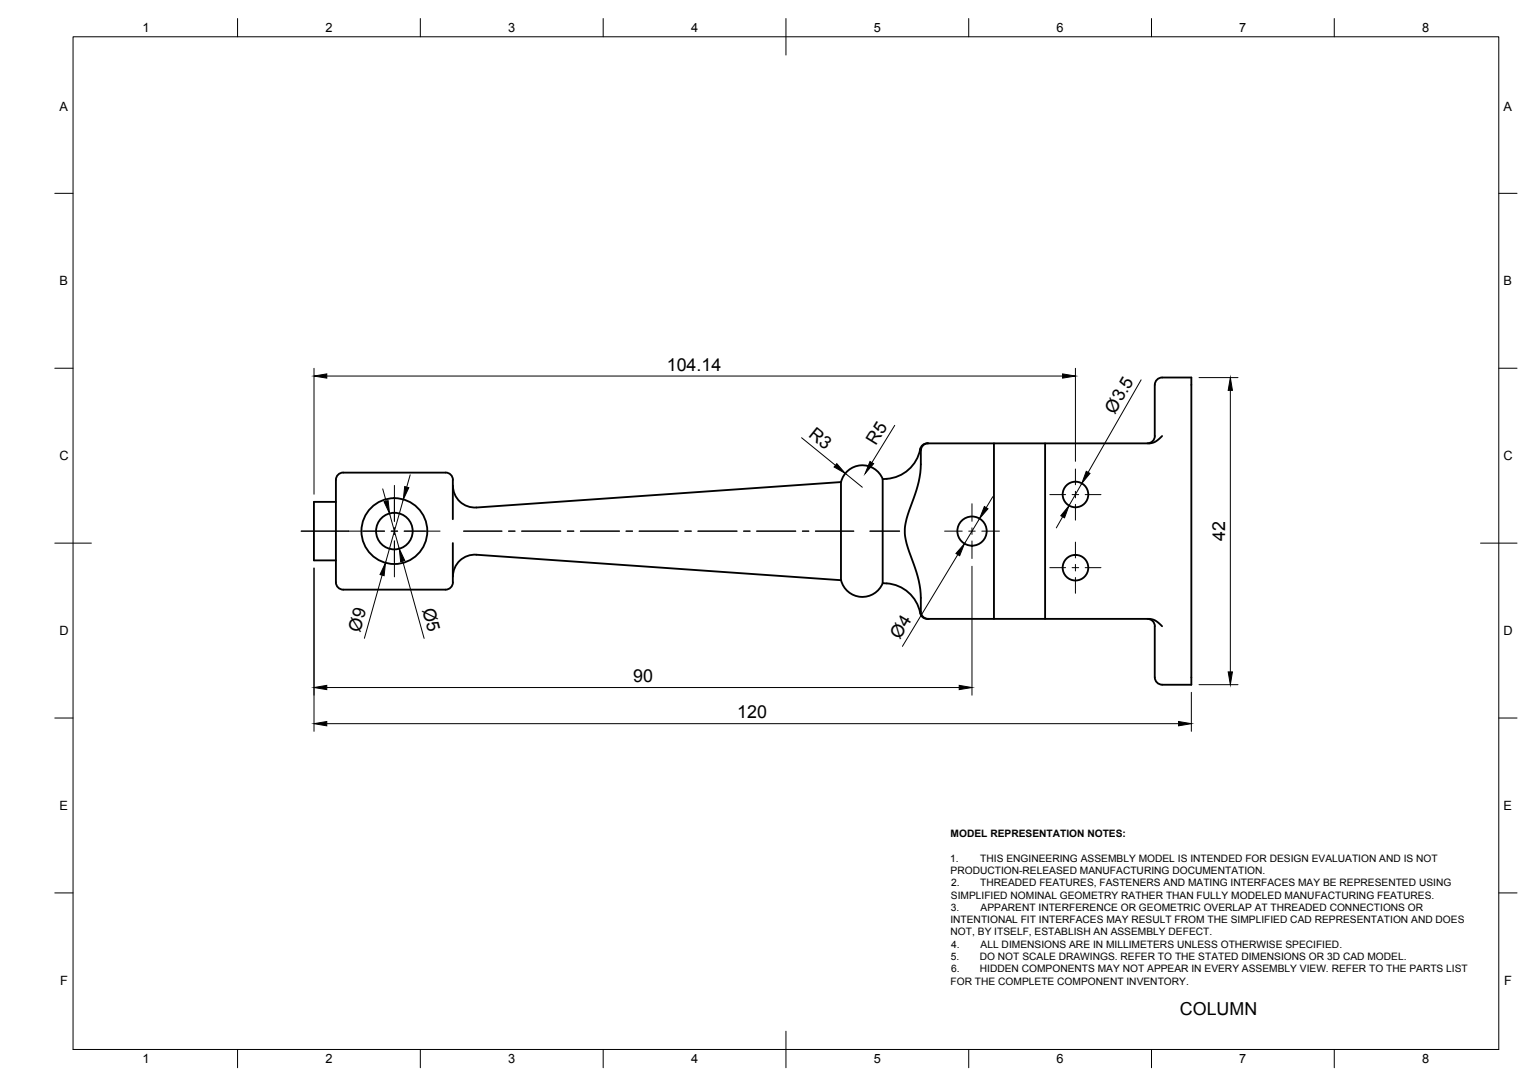
ISO-10303-21;
HEADER;
/* Generated by software containing ST-Developer
 * from STEP Tools, Inc. (www.steptools.com) 
 */

FILE_DESCRIPTION(
/* description */ (''),
/* implementation_level */ '2;1');

FILE_NAME(
/* name */ 'COLUMN.step',
/* time_stamp */ '2026-10-06T01:16:10-07:00',
/* author */ (''),
/* organization */ (''),
/* preprocessor_version */ 'ST-DEVELOPER v20.2',
/* originating_system */ 'Autodesk Translation Framework v15.15.0.0',
/* authorisation */ '');

FILE_SCHEMA (('AUTOMOTIVE_DESIGN { 1 0 10303 214 3 1 1 }'));
ENDSEC;

DATA;
#10=MECHANICAL_DESIGN_GEOMETRIC_PRESENTATION_REPRESENTATION('',(#300,#301,#302),#17113);
#105=ELLIPSE('',#6445,1.4142135623731,1.);
#106=ELLIPSE('',#6457,1.41421356237309,1.);
#109=(
BOUNDED_SURFACE()
B_SPLINE_SURFACE(3,3,((#9243,#9244,#9245,#9246,#9247,#9248,#9249,#9250,
#9251,#9252,#9253,#9254,#9255),(#9256,#9257,#9258,#9259,#9260,#9261,#9262,
#9263,#9264,#9265,#9266,#9267,#9268),(#9269,#9270,#9271,#9272,#9273,#9274,
#9275,#9276,#9277,#9278,#9279,#9280,#9281),(#9282,#9283,#9284,#9285,#9286,
#9287,#9288,#9289,#9290,#9291,#9292,#9293,#9294)),.UNSPECIFIED.,.F.,.F.,
 .F.)
B_SPLINE_SURFACE_WITH_KNOTS((4,4),(4,1,1,1,1,1,1,1,1,1,4),(0.,1.),(-0.01854087386661,
0.,0.124538046056,0.2354380828125,0.3411963661322,0.4510248812945,0.5701285898783,
0.7002368466242,0.8429884965965,1.,1.018551127109),.UNSPECIFIED.)
GEOMETRIC_REPRESENTATION_ITEM()
RATIONAL_B_SPLINE_SURFACE(((1.236576476327,1.236576476327,1.236576476327,
1.236576476327,1.236576476327,1.236576476327,1.236576476327,1.236576476327,
1.236576476327,1.236576476327,1.236576476327,1.236576476327,1.236576476327),
(0.9211411745578,0.9211411745578,0.9211411745578,0.9211411745578,0.9211411745578,
0.9211411745578,0.9211411745578,0.9211411745578,0.9211411745578,0.9211411745578,
0.9211411745578,0.9211411745578,0.9211411745578),(0.9211411745578,0.9211411745578,
0.9211411745578,0.9211411745578,0.9211411745578,0.9211411745578,0.9211411745578,
0.9211411745578,0.9211411745578,0.9211411745578,0.9211411745578,0.9211411745578,
0.9211411745578),(1.236576476327,1.236576476327,1.236576476327,1.236576476327,
1.236576476327,1.236576476327,1.236576476327,1.236576476327,1.236576476327,
1.236576476327,1.236576476327,1.236576476327,1.236576476327)))
REPRESENTATION_ITEM('')
SURFACE()
);
#110=(
BOUNDED_SURFACE()
B_SPLINE_SURFACE(3,3,((#9423,#9424,#9425,#9426,#9427,#9428,#9429,#9430,
#9431,#9432,#9433,#9434,#9435),(#9436,#9437,#9438,#9439,#9440,#9441,#9442,
#9443,#9444,#9445,#9446,#9447,#9448),(#9449,#9450,#9451,#9452,#9453,#9454,
#9455,#9456,#9457,#9458,#9459,#9460,#9461),(#9462,#9463,#9464,#9465,#9466,
#9467,#9468,#9469,#9470,#9471,#9472,#9473,#9474)),.UNSPECIFIED.,.F.,.F.,
 .F.)
B_SPLINE_SURFACE_WITH_KNOTS((4,4),(4,1,1,1,1,1,1,1,1,1,4),(0.,1.),(-0.01854087386661,
0.,0.124538046056,0.2354380828125,0.3411963661322,0.4510248812945,0.5701285898783,
0.7002368466242,0.8429884965965,1.,1.018551127109),.UNSPECIFIED.)
GEOMETRIC_REPRESENTATION_ITEM()
RATIONAL_B_SPLINE_SURFACE(((1.236576476327,1.236576476327,1.236576476327,
1.236576476327,1.236576476327,1.236576476327,1.236576476327,1.236576476327,
1.236576476327,1.236576476327,1.236576476327,1.236576476327,1.236576476327),
(0.9211411745578,0.9211411745578,0.9211411745578,0.9211411745578,0.9211411745578,
0.9211411745578,0.9211411745578,0.9211411745578,0.9211411745578,0.9211411745578,
0.9211411745578,0.9211411745578,0.9211411745578),(0.9211411745578,0.9211411745578,
0.9211411745578,0.9211411745578,0.9211411745578,0.9211411745578,0.9211411745578,
0.9211411745578,0.9211411745578,0.9211411745578,0.9211411745578,0.9211411745578,
0.9211411745578),(1.236576476327,1.236576476327,1.236576476327,1.236576476327,
1.236576476327,1.236576476327,1.236576476327,1.236576476327,1.236576476327,
1.236576476327,1.236576476327,1.236576476327,1.236576476327)))
REPRESENTATION_ITEM('')
SURFACE()
);
#111=(
BOUNDED_SURFACE()
B_SPLINE_SURFACE(3,3,((#9791,#9792,#9793,#9794,#9795,#9796,#9797,#9798,
#9799,#9800,#9801,#9802,#9803,#9804,#9805,#9806,#9807),(#9808,#9809,#9810,
#9811,#9812,#9813,#9814,#9815,#9816,#9817,#9818,#9819,#9820,#9821,#9822,
#9823,#9824),(#9825,#9826,#9827,#9828,#9829,#9830,#9831,#9832,#9833,#9834,
#9835,#9836,#9837,#9838,#9839,#9840,#9841),(#9842,#9843,#9844,#9845,#9846,
#9847,#9848,#9849,#9850,#9851,#9852,#9853,#9854,#9855,#9856,#9857,#9858)),
 .UNSPECIFIED.,.F.,.F.,.F.)
B_SPLINE_SURFACE_WITH_KNOTS((4,4),(4,1,1,1,1,1,1,1,1,1,1,1,1,1,4),(0.,1.),
(-0.009903506240665,0.,0.09441816002876,0.1881578788494,0.280939071815,
0.3715247502583,0.4641517260557,0.5619785611963,0.6570408645664,0.7414898315922,
0.8160167895793,0.8826179898193,0.9432826185749,1.,1.009908876933),
 .UNSPECIFIED.)
GEOMETRIC_REPRESENTATION_ITEM()
RATIONAL_B_SPLINE_SURFACE(((1.236576619558,1.236576619558,1.236576619558,
1.236576619558,1.236576619558,1.236576619558,1.236576619558,1.236576619558,
1.236576619558,1.236576619558,1.236576619558,1.236576619558,1.236576619558,
1.236576619558,1.236576619558,1.236576619558,1.236576619558),(0.9211411268139,
0.9211411268139,0.9211411268139,0.9211411268139,0.9211411268139,0.9211411268139,
0.9211411268139,0.9211411268139,0.9211411268139,0.9211411268139,0.9211411268139,
0.9211411268139,0.9211411268139,0.9211411268139,0.9211411268139,0.9211411268139,
0.9211411268139),(0.9211411268139,0.9211411268139,0.9211411268139,0.9211411268139,
0.9211411268139,0.9211411268139,0.9211411268139,0.9211411268139,0.9211411268139,
0.9211411268139,0.9211411268139,0.9211411268139,0.9211411268139,0.9211411268139,
0.9211411268139,0.9211411268139,0.9211411268139),(1.236576619558,1.236576619558,
1.236576619558,1.236576619558,1.236576619558,1.236576619558,1.236576619558,
1.236576619558,1.236576619558,1.236576619558,1.236576619558,1.236576619558,
1.236576619558,1.236576619558,1.236576619558,1.236576619558,1.236576619558)))
REPRESENTATION_ITEM('')
SURFACE()
);
#112=(
BOUNDED_SURFACE()
B_SPLINE_SURFACE(3,3,((#10155,#10156,#10157,#10158,#10159,#10160,#10161,
#10162,#10163,#10164,#10165),(#10166,#10167,#10168,#10169,#10170,#10171,
#10172,#10173,#10174,#10175,#10176),(#10177,#10178,#10179,#10180,#10181,
#10182,#10183,#10184,#10185,#10186,#10187),(#10188,#10189,#10190,#10191,
#10192,#10193,#10194,#10195,#10196,#10197,#10198)),.UNSPECIFIED.,.F.,.F.,
 .F.)
B_SPLINE_SURFACE_WITH_KNOTS((4,4),(4,1,1,1,1,1,1,1,4),(0.,1.),(-0.0117961357116,
0.,0.1633770608974,0.3160773256608,0.4701362865974,0.6315432333968,0.8054144885927,
1.,1.011975292336),.UNSPECIFIED.)
GEOMETRIC_REPRESENTATION_ITEM()
RATIONAL_B_SPLINE_SURFACE(((1.236576493506,1.236576493506,1.236576493506,
1.236576493506,1.236576493506,1.236576493506,1.236576493506,1.236576493506,
1.236576493506,1.236576493506,1.236576493506),(0.9211411688312,0.9211411688312,
0.9211411688312,0.9211411688312,0.9211411688312,0.9211411688312,0.9211411688312,
0.9211411688312,0.9211411688312,0.9211411688312,0.9211411688312),(0.9211411688312,
0.9211411688312,0.9211411688312,0.9211411688312,0.9211411688312,0.9211411688312,
0.9211411688312,0.9211411688312,0.9211411688312,0.9211411688312,0.9211411688312),
(1.236576493506,1.236576493506,1.236576493506,1.236576493506,1.236576493506,
1.236576493506,1.236576493506,1.236576493506,1.236576493506,1.236576493506,
1.236576493506)))
REPRESENTATION_ITEM('')
SURFACE()
);
#113=(
BOUNDED_SURFACE()
B_SPLINE_SURFACE(3,3,((#10200,#10201,#10202,#10203,#10204,#10205,#10206,
#10207,#10208,#10209,#10210,#10211,#10212),(#10213,#10214,#10215,#10216,
#10217,#10218,#10219,#10220,#10221,#10222,#10223,#10224,#10225),(#10226,
#10227,#10228,#10229,#10230,#10231,#10232,#10233,#10234,#10235,#10236,#10237,
#10238),(#10239,#10240,#10241,#10242,#10243,#10244,#10245,#10246,#10247,
#10248,#10249,#10250,#10251)),.UNSPECIFIED.,.F.,.F.,.F.)
B_SPLINE_SURFACE_WITH_KNOTS((4,4),(4,1,1,1,1,1,1,1,1,1,4),(0.,1.),(-0.02387271189713,
0.,0.1233219598256,0.2447228034141,0.3668475159477,0.4855515195745,0.6022629448181,
0.7239422574426,0.8555602069799,1.,1.011825585123),.UNSPECIFIED.)
GEOMETRIC_REPRESENTATION_ITEM()
RATIONAL_B_SPLINE_SURFACE(((1.236576471212,1.236576471212,1.236576471212,
1.236576471212,1.236576471212,1.236576471212,1.236576471212,1.236576471212,
1.236576471212,1.236576471212,1.236576471212,1.236576471212,1.236576471212),
(0.9211411762628,0.9211411762628,0.9211411762628,0.9211411762628,0.9211411762628,
0.9211411762628,0.9211411762628,0.9211411762628,0.9211411762628,0.9211411762628,
0.9211411762628,0.9211411762628,0.9211411762628),(0.9211411762628,0.9211411762628,
0.9211411762628,0.9211411762628,0.9211411762628,0.9211411762628,0.9211411762628,
0.9211411762628,0.9211411762628,0.9211411762628,0.9211411762628,0.9211411762628,
0.9211411762628),(1.236576471212,1.236576471212,1.236576471212,1.236576471212,
1.236576471212,1.236576471212,1.236576471212,1.236576471212,1.236576471212,
1.236576471212,1.236576471212,1.236576471212,1.236576471212)))
REPRESENTATION_ITEM('')
SURFACE()
);
#114=SPHERICAL_SURFACE('',#6330,1.);
#115=SPHERICAL_SURFACE('',#6351,1.);
#116=SPHERICAL_SURFACE('',#6354,1.);
#117=SPHERICAL_SURFACE('',#6359,1.);
#118=SPHERICAL_SURFACE('',#6367,1.);
#119=SPHERICAL_SURFACE('',#6371,1.);
#120=SPHERICAL_SURFACE('',#6382,1.);
#121=SPHERICAL_SURFACE('',#6383,1.);
#122=SPHERICAL_SURFACE('',#6480,1.);
#123=SPHERICAL_SURFACE('',#6487,1.);
#124=SPHERICAL_SURFACE('',#6499,1.);
#125=SPHERICAL_SURFACE('',#6505,1.);
#126=TOROIDAL_SURFACE('',#6307,4.,0.5);
#127=TOROIDAL_SURFACE('',#6316,4.,0.5);
#128=TOROIDAL_SURFACE('',#6343,6.217106130074,3.);
#129=TOROIDAL_SURFACE('',#6401,6.,3.);
#130=TOROIDAL_SURFACE('',#6403,12.13789139507,5.);
#131=TOROIDAL_SURFACE('',#6435,2.,1.);
#132=TOROIDAL_SURFACE('',#6459,2.,1.);
#133=TOROIDAL_SURFACE('',#6492,2.,1.);
#134=TOROIDAL_SURFACE('',#6509,2.,1.);
#146=B_SPLINE_CURVE_WITH_KNOTS('',3,(#9111,#9112,#9113,#9114,#9115,#9116,
#9117,#9118,#9119,#9120,#9121),.UNSPECIFIED.,.F.,.F.,(4,1,1,1,1,1,1,1,4),
(5.02030750257932E-6,0.125,0.25,0.375,0.5,0.625,0.75,0.875,1.),
 .UNSPECIFIED.);
#147=B_SPLINE_CURVE_WITH_KNOTS('',3,(#9146,#9147,#9148,#9149,#9150,#9151,
#9152,#9153,#9154,#9155,#9156,#9157,#9158,#9159,#9160,#9161,#9162,#9163),
 .UNSPECIFIED.,.F.,.F.,(4,2,2,2,2,2,2,2,4),(0.38439055210377,0.432504952213954,
0.480619352324138,0.528602590239896,0.576585828155655,0.624569066071413,
0.672552303987171,0.720666704097356,0.76878110420754),.UNSPECIFIED.);
#148=B_SPLINE_CURVE_WITH_KNOTS('',3,(#9164,#9165,#9166,#9167,#9168,#9169,
#9170,#9171,#9172,#9173,#9174,#9175,#9176,#9177,#9178,#9179,#9180,#9181),
 .UNSPECIFIED.,.F.,.F.,(4,2,2,2,2,2,2,2,4),(0.76878110420754,0.816895504317724,
0.865009904427908,0.912993142343666,0.960976380259425,1.00895961817518,
1.05694285609094,1.10505725620113,1.15317165631131),.UNSPECIFIED.);
#149=B_SPLINE_CURVE_WITH_KNOTS('',3,(#9206,#9207,#9208,#9209,#9210,#9211,
#9212,#9213,#9214,#9215,#9216),.UNSPECIFIED.,.F.,.F.,(4,1,1,1,1,1,1,1,4),
(5.02030750249862E-6,0.125,0.25,0.375,0.5,0.625,0.75,0.875,1.),
 .UNSPECIFIED.);
#150=B_SPLINE_CURVE_WITH_KNOTS('',3,(#9296,#9297,#9298,#9299,#9300,#9301,
#9302,#9303,#9304,#9305,#9306,#9307,#9308,#9309,#9310,#9311,#9312,#9313,
#9314,#9315,#9316,#9317,#9318,#9319,#9320,#9321,#9322,#9323,#9324,#9325,
#9326,#9327,#9328,#9329,#9330,#9331,#9332,#9333,#9334,#9335,#9336,#9337,
#9338,#9339,#9340,#9341,#9342,#9343,#9344),.UNSPECIFIED.,.F.,.F.,(4,3,3,
3,3,3,3,3,3,3,3,3,3,3,3,3,4),(4.37386987750375E-6,0.0927050507258515,0.125,
0.21480736126803,0.25,0.35993980774069,0.375,0.491161389173609,0.5,0.611281050311693,
0.625,0.72687460423662,0.75,0.841555339636589,0.875,0.952466785368161,1.),
 .UNSPECIFIED.);
#151=B_SPLINE_CURVE_WITH_KNOTS('',3,(#9368,#9369,#9370,#9371,#9372,#9373,
#9374,#9375,#9376,#9377,#9378,#9379,#9380,#9381,#9382,#9383,#9384,#9385,
#9386,#9387,#9388,#9389,#9390,#9391,#9392,#9393,#9394,#9395,#9396,#9397,
#9398,#9399,#9400,#9401,#9402,#9403,#9404,#9405,#9406,#9407,#9408,#9409,
#9410,#9411,#9412,#9413,#9414,#9415,#9416,#9417,#9418,#9419,#9420,#9421,
#9422),.UNSPECIFIED.,.F.,.F.,(4,3,3,3,3,3,3,3,3,3,3,3,3,3,3,3,3,3,4),(4.37386990229217E-6,
0.078116780989183,0.125,0.178786314155506,0.234096638055846,0.25,0.307075966738911,
0.364185364927029,0.375,0.440633200921451,0.5,0.585859467132409,0.625,0.699968906702808,
0.75,0.824334220487127,0.875,0.940179003774522,1.),.UNSPECIFIED.);
#152=B_SPLINE_CURVE_WITH_KNOTS('',3,(#9566,#9567,#9568,#9569,#9570,#9571,
#9572,#9573,#9574,#9575),.UNSPECIFIED.,.F.,.F.,(4,2,2,2,4),(5.976817519871,
6.14313994502015,6.3094623701693,6.59082757274907,6.87100413233151),
 .UNSPECIFIED.);
#153=B_SPLINE_CURVE_WITH_KNOTS('',3,(#9579,#9580,#9581,#9582,#9583,#9584,
#9585,#9586,#9587,#9588,#9589,#9590,#9591,#9592,#9593,#9594,#9595,#9596,
#9597,#9598,#9599,#9600,#9601,#9602,#9603,#9604,#9605,#9606,#9607,#9608,
#9609,#9610,#9611,#9612,#9613,#9614,#9615,#9616,#9617,#9618,#9619,#9620,
#9621),.UNSPECIFIED.,.F.,.F.,(4,3,3,3,3,3,3,3,3,3,3,3,3,3,4),(4.15972417351908E-9,
0.0998336668422238,0.1666666666667,0.243344677320033,0.328047736632198,
0.3333333333333,0.448940244692513,0.5,0.600185553237847,0.6666666666667,
0.75,0.825496133016552,0.8333333333333,0.92981319294891,0.999999999596363),
 .UNSPECIFIED.);
#154=B_SPLINE_CURVE_WITH_KNOTS('',3,(#9623,#9624,#9625,#9626,#9627,#9628,
#9629,#9630,#9631,#9632,#9633,#9634,#9635,#9636,#9637,#9638,#9639,#9640,
#9641,#9642,#9643,#9644,#9645,#9646,#9647,#9648,#9649,#9650,#9651,#9652,
#9653,#9654,#9655,#9656,#9657,#9658,#9659,#9660,#9661,#9662,#9663,#9664,
#9665,#9666,#9667,#9668),.UNSPECIFIED.,.F.,.F.,(4,3,3,3,3,3,3,3,3,3,3,3,
3,3,3,4),(0.,0.125,0.210638947521259,0.25,0.337872505342455,0.375,0.480596631880562,
0.5,0.597224358508775,0.625,0.710418048307479,0.75,0.823358228203642,0.875,
0.94278763723167,0.999999999303434),.UNSPECIFIED.);
#155=B_SPLINE_CURVE_WITH_KNOTS('',3,(#9672,#9673,#9674,#9675,#9676,#9677,
#9678,#9679,#9680,#9681,#9682,#9683,#9684,#9685,#9686,#9687,#9688,#9689,
#9690),.UNSPECIFIED.,.F.,.F.,(4,2,2,2,3,2,2,2,4),(-0.895375255457832,-0.72905283030868,
-0.562730405159529,-0.281365202579764,0.,0.281365202579765,0.562730405159529,
0.729052830308681,0.895375255457832),.UNSPECIFIED.);
#156=B_SPLINE_CURVE_WITH_KNOTS('',3,(#9694,#9695,#9696,#9697,#9698,#9699,
#9700,#9701,#9702,#9703,#9704,#9705,#9706,#9707,#9708,#9709,#9710,#9711,
#9712,#9713,#9714,#9715,#9716,#9717,#9718,#9719,#9720,#9721,#9722,#9723,
#9724,#9725,#9726,#9727,#9728,#9729,#9730,#9731,#9732,#9733,#9734,#9735,
#9736,#9737,#9738,#9739,#9740,#9741,#9742,#9743,#9744,#9745,#9746,#9747,
#9748,#9749,#9750,#9751,#9752,#9753,#9754,#9755,#9756,#9757,#9758,#9759,
#9760,#9761,#9762,#9763,#9764,#9765,#9766,#9767,#9768,#9769,#9770,#9771,
#9772,#9773,#9774,#9775),.UNSPECIFIED.,.F.,.F.,(4,3,3,3,3,3,3,3,3,3,3,3,
3,3,3,3,3,3,3,3,3,3,3,3,3,3,3,4),(0.,0.0559513285251171,0.08333333333333,
0.1666666666667,0.216931260660868,0.25,0.294848169718225,0.3333333333333,
0.375,0.413940896871108,0.4166666666667,0.451751192947467,0.486849107740909,
0.5,0.53799564679006,0.577957191404146,0.5833333333333,0.622184542089551,
0.663983458717584,0.6666666666667,0.712268138213338,0.75,0.801593987292321,
0.8333333333333,0.893036722145433,0.9166666666667,0.97337992594817,0.999999974018396),
 .UNSPECIFIED.);
#157=B_SPLINE_CURVE_WITH_KNOTS('',3,(#9778,#9779,#9780,#9781,#9782,#9783,
#9784,#9785,#9786,#9787,#9788,#9789,#9790),.UNSPECIFIED.,.F.,.F.,(4,3,2,
2,2,4),(6.87100413233151,6.87219277532883,7.1535579779086,7.43492318048836,
7.60124560563752,7.76756803078667),.UNSPECIFIED.);
#158=B_SPLINE_CURVE_WITH_KNOTS('',3,(#9861,#9862,#9863,#9864,#9865,#9866,
#9867,#9868,#9869,#9870,#9871,#9872,#9873,#9874,#9875),.UNSPECIFIED.,.F.,
 .F.,(4,1,1,1,1,1,1,1,1,1,1,1,4),(4.80530147585308E-8,0.08333333333333,
0.1666666666667,0.25,0.3333333333333,0.4166666666667,0.5,0.5833333333333,
0.6666666666667,0.75,0.8333333333333,0.9166666666667,0.999999273982094),
 .UNSPECIFIED.);
#159=B_SPLINE_CURVE_WITH_KNOTS('',3,(#9904,#9905,#9906,#9907),
 .UNSPECIFIED.,.F.,.F.,(4,4),(0.779469865639367,0.833309307571144),
 .UNSPECIFIED.);
#160=B_SPLINE_CURVE_WITH_KNOTS('',3,(#9909,#9910,#9911,#9912,#9913,#9914,
#9915,#9916,#9917,#9918,#9919,#9920,#9921,#9922,#9923,#9924,#9925,#9926,
#9927,#9928,#9929,#9930,#9931,#9932,#9933),.UNSPECIFIED.,.F.,.F.,(4,2,2,
2,2,3,2,2,2,2,2,4),(0.833309307571144,0.908998418331253,0.984687529091362,
1.05819154321553,1.09494355027761,1.13169555733969,1.16844756440177,1.20519957146385,
1.27870358558802,1.35439269634812,1.43008180710823,1.48392124906823),
 .UNSPECIFIED.);
#161=B_SPLINE_CURVE_WITH_KNOTS('',3,(#9937,#9938,#9939,#9940,#9941,#9942,
#9943,#9944,#9945,#9946,#9947,#9948,#9949,#9950,#9951,#9952,#9953,#9954),
 .UNSPECIFIED.,.F.,.F.,(4,2,2,2,2,2,2,2,4),(0.352225691728541,0.364327757248449,
0.430269264728352,0.498058521699098,0.565847778669844,0.63363703564059,
0.701426292611336,0.76736780009124,0.779469865639367),.UNSPECIFIED.);
#162=B_SPLINE_CURVE_WITH_KNOTS('',3,(#9979,#9980,#9981,#9982,#9983,#9984),
 .UNSPECIFIED.,.F.,.F.,(4,2,4),(0.,0.117562819132916,0.19402604569559),
 .UNSPECIFIED.);
#163=B_SPLINE_CURVE_WITH_KNOTS('',3,(#9995,#9996,#9997,#9998,#9999,#10000),
 .UNSPECIFIED.,.F.,.F.,(4,2,4),(0.505532240038497,0.581995466601172,0.699558285734087),
 .UNSPECIFIED.);
#164=B_SPLINE_CURVE_WITH_KNOTS('',3,(#10006,#10007,#10008,#10009,#10010,
#10011,#10012,#10013,#10014,#10015,#10016,#10017,#10018,#10019,#10020,#10021,
#10022,#10023,#10024,#10025,#10026,#10027,#10028),.UNSPECIFIED.,.F.,.F.,
(4,2,2,2,2,3,2,2,2,2,4),(0.833309307571144,0.908998418331253,0.984687529091362,
1.05819154321553,1.09494355027761,1.13169555733969,1.16844756440177,1.20519957146385,
1.27870358558802,1.35439269634812,1.43008180710823),.UNSPECIFIED.);
#165=B_SPLINE_CURVE_WITH_KNOTS('',3,(#10031,#10032,#10033,#10034),
 .UNSPECIFIED.,.F.,.F.,(4,4),(1.43008180710823,1.48392124904001),
 .UNSPECIFIED.);
#166=B_SPLINE_CURVE_WITH_KNOTS('',3,(#10036,#10037,#10038,#10039,#10040,
#10041,#10042,#10043,#10044,#10045,#10046,#10047,#10048,#10049,#10050,#10051,
#10052,#10053),.UNSPECIFIED.,.F.,.F.,(4,2,2,2,2,2,2,2,4),(1.48392124904001,
1.49602331458814,1.56196482206804,1.62975407903879,1.69754333600953,1.76533259298028,
1.83312184995102,1.89906335743093,1.91116542297906),.UNSPECIFIED.);
#167=B_SPLINE_CURVE_WITH_KNOTS('',3,(#10054,#10055,#10056,#10057),
 .UNSPECIFIED.,.F.,.F.,(4,4),(1.91116542297906,1.96500486491083),
 .UNSPECIFIED.);
#168=B_SPLINE_CURVE_WITH_KNOTS('',3,(#10074,#10075,#10076,#10077,#10078,
#10079,#10080,#10081,#10082,#10083,#10084),.UNSPECIFIED.,.F.,.F.,(4,1,1,
1,1,1,1,1,4),(0.,0.125,0.25,0.375,0.5,0.625,0.75,0.875,0.999999972808484),
 .UNSPECIFIED.);
#169=B_SPLINE_CURVE_WITH_KNOTS('',3,(#10086,#10087,#10088,#10089,#10090,
#10091,#10092,#10093,#10094),.UNSPECIFIED.,.F.,.F.,(4,1,1,1,1,1,4),(1.77479359457994E-7,
0.1666666666667,0.3333333333333,0.5,0.6666666666667,0.8333333333333,1.),
 .UNSPECIFIED.);
#223=OPEN_SHELL('',(#5804,#5805));
#224=OPEN_SHELL('',(#5806,#5807));
#241=SHELL_BASED_SURFACE_MODEL('Body2',(#223));
#242=SHELL_BASED_SURFACE_MODEL('Body3',(#224));
#261=CONICAL_SURFACE('',#6390,1.375,0.785398163397448);
#262=CONICAL_SURFACE('',#6393,5.187242561534,0.0698131700797732);
#263=CONICAL_SURFACE('',#6396,5.187242561534,0.0698131700797732);
#266=SHAPE_REPRESENTATION_RELATIONSHIP('SRR','None',#17188,#282);
#282=ADVANCED_BREP_SHAPE_REPRESENTATION('',(#332),#17095);
#300=STYLED_ITEM('',(#17298),#332);
#301=STYLED_ITEM('',(#17298),#241);
#302=STYLED_ITEM('',(#17298),#242);
#332=MANIFOLD_SOLID_BREP('Body1',#6018);
#364=CYLINDRICAL_SURFACE('',#6304,4.5);
#365=CYLINDRICAL_SURFACE('',#6312,2.5);
#366=CYLINDRICAL_SURFACE('',#6320,4.5);
#367=CYLINDRICAL_SURFACE('',#6323,1.);
#368=CYLINDRICAL_SURFACE('',#6327,1.);
#369=CYLINDRICAL_SURFACE('',#6333,1.);
#370=CYLINDRICAL_SURFACE('',#6336,1.);
#371=CYLINDRICAL_SURFACE('',#6349,1.);
#372=CYLINDRICAL_SURFACE('',#6352,1.);
#373=CYLINDRICAL_SURFACE('',#6357,1.);
#374=CYLINDRICAL_SURFACE('',#6361,1.);
#375=CYLINDRICAL_SURFACE('',#6364,1.);
#376=CYLINDRICAL_SURFACE('',#6369,1.);
#377=CYLINDRICAL_SURFACE('',#6374,1.);
#378=CYLINDRICAL_SURFACE('',#6375,1.);
#379=CYLINDRICAL_SURFACE('',#6379,1.);
#380=CYLINDRICAL_SURFACE('',#6385,1.);
#381=CYLINDRICAL_SURFACE('',#6386,4.);
#382=CYLINDRICAL_SURFACE('',#6392,1.25);
#383=CYLINDRICAL_SURFACE('',#6414,2.625);
#384=CYLINDRICAL_SURFACE('',#6417,1.75);
#385=CYLINDRICAL_SURFACE('',#6425,1.75);
#386=CYLINDRICAL_SURFACE('',#6426,2.625);
#387=CYLINDRICAL_SURFACE('',#6432,1.);
#388=CYLINDRICAL_SURFACE('',#6442,2.);
#389=CYLINDRICAL_SURFACE('',#6443,1.);
#390=CYLINDRICAL_SURFACE('',#6446,1.);
#391=CYLINDRICAL_SURFACE('',#6451,1.);
#392=CYLINDRICAL_SURFACE('',#6452,1.);
#393=CYLINDRICAL_SURFACE('',#6456,1.);
#394=CYLINDRICAL_SURFACE('',#6458,1.);
#395=CYLINDRICAL_SURFACE('',#6462,1.);
#396=CYLINDRICAL_SURFACE('',#6467,2.);
#397=CYLINDRICAL_SURFACE('',#6475,2.);
#398=CYLINDRICAL_SURFACE('',#6478,1.);
#399=CYLINDRICAL_SURFACE('',#6483,1.);
#400=CYLINDRICAL_SURFACE('',#6485,1.);
#401=CYLINDRICAL_SURFACE('',#6490,1.);
#402=CYLINDRICAL_SURFACE('',#6493,1.);
#403=CYLINDRICAL_SURFACE('',#6494,1.);
#404=CYLINDRICAL_SURFACE('',#6497,1.);
#405=CYLINDRICAL_SURFACE('',#6502,1.);
#406=CYLINDRICAL_SURFACE('',#6503,1.);
#407=CYLINDRICAL_SURFACE('',#6507,1.);
#408=CYLINDRICAL_SURFACE('',#6513,3.);
#409=CYLINDRICAL_SURFACE('',#6518,3.);
#528=FACE_BOUND('',#1439,.T.);
#529=FACE_BOUND('',#1443,.T.);
#530=FACE_BOUND('',#1445,.T.);
#531=FACE_BOUND('',#1447,.T.);
#532=FACE_BOUND('',#1451,.T.);
#533=FACE_BOUND('',#1478,.T.);
#534=FACE_BOUND('',#1485,.T.);
#535=FACE_BOUND('',#1494,.T.);
#536=FACE_BOUND('',#1499,.T.);
#537=FACE_BOUND('',#1501,.T.);
#538=FACE_BOUND('',#1502,.T.);
#539=FACE_BOUND('',#1506,.T.);
#540=FACE_BOUND('',#1511,.T.);
#541=FACE_BOUND('',#1530,.T.);
#542=FACE_BOUND('',#1531,.T.);
#543=FACE_BOUND('',#1557,.T.);
#544=FACE_BOUND('',#1560,.T.);
#678=CIRCLE('',#6303,4.5);
#679=CIRCLE('',#6305,4.5);
#680=CIRCLE('',#6306,4.5);
#681=CIRCLE('',#6308,0.5);
#682=CIRCLE('',#6309,4.);
#683=CIRCLE('',#6311,2.5);
#684=CIRCLE('',#6313,2.5);
#685=CIRCLE('',#6315,4.);
#686=CIRCLE('',#6317,0.5);
#687=CIRCLE('',#6318,4.5);
#688=CIRCLE('',#6319,4.5);
#689=CIRCLE('',#6321,4.5);
#690=CIRCLE('',#6324,1.);
#691=CIRCLE('',#6325,1.);
#692=CIRCLE('',#6328,1.);
#693=CIRCLE('',#6329,1.);
#694=CIRCLE('',#6331,1.);
#695=CIRCLE('',#6332,1.);
#696=CIRCLE('',#6334,1.);
#697=CIRCLE('',#6335,1.);
#698=CIRCLE('',#6337,1.);
#699=CIRCLE('',#6339,6.217106130074);
#700=CIRCLE('',#6340,6.217106130074);
#701=CIRCLE('',#6342,6.217106130074);
#702=CIRCLE('',#6344,3.);
#703=CIRCLE('',#6345,3.224413979295);
#704=CIRCLE('',#6346,3.224413979295);
#705=CIRCLE('',#6347,1.);
#706=CIRCLE('',#6348,1.);
#707=CIRCLE('',#6350,1.);
#708=CIRCLE('',#6353,1.);
#709=CIRCLE('',#6355,1.);
#710=CIRCLE('',#6356,1.);
#711=CIRCLE('',#6358,1.);
#712=CIRCLE('',#6360,1.);
#713=CIRCLE('',#6362,1.);
#714=CIRCLE('',#6365,1.);
#715=CIRCLE('',#6366,1.);
#716=CIRCLE('',#6368,1.);
#717=CIRCLE('',#6370,1.);
#718=CIRCLE('',#6372,1.);
#719=CIRCLE('',#6373,1.);
#720=CIRCLE('',#6376,1.);
#721=CIRCLE('',#6378,4.);
#722=CIRCLE('',#6380,1.);
#723=CIRCLE('',#6381,1.);
#724=CIRCLE('',#6384,1.);
#725=CIRCLE('',#6387,4.);
#726=CIRCLE('',#6389,1.5);
#727=CIRCLE('',#6391,1.25);
#728=CIRCLE('',#6394,6.712116818331);
#729=CIRCLE('',#6395,6.712116818331);
#730=CIRCLE('',#6397,7.150071143774);
#731=CIRCLE('',#6398,7.150071143774);
#732=CIRCLE('',#6399,7.110772629208);
#733=CIRCLE('',#6400,7.110772629208);
#734=CIRCLE('',#6402,3.);
#735=CIRCLE('',#6404,5.);
#736=CIRCLE('',#6405,12.13789139507);
#737=CIRCLE('',#6406,12.13789139507);
#738=CIRCLE('',#6407,12.13789139507);
#739=CIRCLE('',#6408,12.13789139507);
#740=CIRCLE('',#6409,1.);
#741=CIRCLE('',#6410,1.);
#742=CIRCLE('',#6412,2.);
#743=CIRCLE('',#6413,2.625);
#744=CIRCLE('',#6415,2.625);
#745=CIRCLE('',#6418,1.75);
#746=CIRCLE('',#6420,1.);
#747=CIRCLE('',#6421,1.);
#748=CIRCLE('',#6422,2.);
#749=CIRCLE('',#6424,1.75);
#750=CIRCLE('',#6427,2.625);
#751=CIRCLE('',#6428,2.625);
#752=CIRCLE('',#6430,2.);
#753=CIRCLE('',#6433,1.);
#754=CIRCLE('',#6434,1.);
#755=CIRCLE('',#6436,2.);
#756=CIRCLE('',#6437,1.);
#757=CIRCLE('',#6438,1.);
#758=CIRCLE('',#6440,2.);
#759=CIRCLE('',#6441,2.);
#760=CIRCLE('',#6444,1.);
#761=CIRCLE('',#6453,1.);
#762=CIRCLE('',#6454,1.);
#763=CIRCLE('',#6455,1.);
#764=CIRCLE('',#6460,1.);
#765=CIRCLE('',#6461,1.);
#766=CIRCLE('',#6463,1.);
#767=CIRCLE('',#6465,2.);
#768=CIRCLE('',#6466,2.);
#769=CIRCLE('',#6468,2.);
#770=CIRCLE('',#6470,1.);
#771=CIRCLE('',#6471,1.);
#772=CIRCLE('',#6472,1.);
#773=CIRCLE('',#6473,1.);
#774=CIRCLE('',#6474,2.);
#775=CIRCLE('',#6476,2.);
#776=CIRCLE('',#6479,1.);
#777=CIRCLE('',#6481,1.);
#778=CIRCLE('',#6482,1.);
#779=CIRCLE('',#6486,1.);
#780=CIRCLE('',#6488,1.);
#781=CIRCLE('',#6489,1.);
#782=CIRCLE('',#6491,1.);
#783=CIRCLE('',#6495,1.);
#784=CIRCLE('',#6498,1.);
#785=CIRCLE('',#6500,1.);
#786=CIRCLE('',#6501,1.);
#787=CIRCLE('',#6504,1.);
#788=CIRCLE('',#6506,1.);
#789=CIRCLE('',#6508,1.);
#790=CIRCLE('',#6514,3.);
#791=CIRCLE('',#6515,3.);
#792=CIRCLE('',#6517,2.625);
#793=CIRCLE('',#6519,3.);
#794=CIRCLE('',#6520,3.);
#795=CIRCLE('',#6522,2.625);
#1054=FACE_OUTER_BOUND('',#1438,.T.);
#1055=FACE_OUTER_BOUND('',#1440,.T.);
#1056=FACE_OUTER_BOUND('',#1441,.T.);
#1057=FACE_OUTER_BOUND('',#1442,.T.);
#1058=FACE_OUTER_BOUND('',#1444,.T.);
#1059=FACE_OUTER_BOUND('',#1446,.T.);
#1060=FACE_OUTER_BOUND('',#1448,.T.);
#1061=FACE_OUTER_BOUND('',#1449,.T.);
#1062=FACE_OUTER_BOUND('',#1450,.T.);
#1063=FACE_OUTER_BOUND('',#1452,.T.);
#1064=FACE_OUTER_BOUND('',#1453,.T.);
#1065=FACE_OUTER_BOUND('',#1454,.T.);
#1066=FACE_OUTER_BOUND('',#1455,.T.);
#1067=FACE_OUTER_BOUND('',#1456,.T.);
#1068=FACE_OUTER_BOUND('',#1457,.T.);
#1069=FACE_OUTER_BOUND('',#1458,.T.);
#1070=FACE_OUTER_BOUND('',#1459,.T.);
#1071=FACE_OUTER_BOUND('',#1460,.T.);
#1072=FACE_OUTER_BOUND('',#1461,.T.);
#1073=FACE_OUTER_BOUND('',#1462,.T.);
#1074=FACE_OUTER_BOUND('',#1463,.T.);
#1075=FACE_OUTER_BOUND('',#1464,.T.);
#1076=FACE_OUTER_BOUND('',#1465,.T.);
#1077=FACE_OUTER_BOUND('',#1466,.T.);
#1078=FACE_OUTER_BOUND('',#1467,.T.);
#1079=FACE_OUTER_BOUND('',#1468,.T.);
#1080=FACE_OUTER_BOUND('',#1469,.T.);
#1081=FACE_OUTER_BOUND('',#1470,.T.);
#1082=FACE_OUTER_BOUND('',#1471,.T.);
#1083=FACE_OUTER_BOUND('',#1472,.T.);
#1084=FACE_OUTER_BOUND('',#1473,.T.);
#1085=FACE_OUTER_BOUND('',#1474,.T.);
#1086=FACE_OUTER_BOUND('',#1475,.T.);
#1087=FACE_OUTER_BOUND('',#1476,.T.);
#1088=FACE_OUTER_BOUND('',#1477,.T.);
#1089=FACE_OUTER_BOUND('',#1479,.T.);
#1090=FACE_OUTER_BOUND('',#1480,.T.);
#1091=FACE_OUTER_BOUND('',#1481,.T.);
#1092=FACE_OUTER_BOUND('',#1482,.T.);
#1093=FACE_OUTER_BOUND('',#1483,.T.);
#1094=FACE_OUTER_BOUND('',#1484,.T.);
#1095=FACE_OUTER_BOUND('',#1486,.T.);
#1096=FACE_OUTER_BOUND('',#1487,.T.);
#1097=FACE_OUTER_BOUND('',#1488,.T.);
#1098=FACE_OUTER_BOUND('',#1489,.T.);
#1099=FACE_OUTER_BOUND('',#1490,.T.);
#1100=FACE_OUTER_BOUND('',#1491,.T.);
#1101=FACE_OUTER_BOUND('',#1492,.T.);
#1102=FACE_OUTER_BOUND('',#1493,.T.);
#1103=FACE_OUTER_BOUND('',#1495,.T.);
#1104=FACE_OUTER_BOUND('',#1496,.T.);
#1105=FACE_OUTER_BOUND('',#1497,.T.);
#1106=FACE_OUTER_BOUND('',#1498,.T.);
#1107=FACE_OUTER_BOUND('',#1500,.T.);
#1108=FACE_OUTER_BOUND('',#1503,.T.);
#1109=FACE_OUTER_BOUND('',#1504,.T.);
#1110=FACE_OUTER_BOUND('',#1505,.T.);
#1111=FACE_OUTER_BOUND('',#1507,.T.);
#1112=FACE_OUTER_BOUND('',#1508,.T.);
#1113=FACE_OUTER_BOUND('',#1509,.T.);
#1114=FACE_OUTER_BOUND('',#1510,.T.);
#1115=FACE_OUTER_BOUND('',#1512,.T.);
#1116=FACE_OUTER_BOUND('',#1513,.T.);
#1117=FACE_OUTER_BOUND('',#1514,.T.);
#1118=FACE_OUTER_BOUND('',#1515,.T.);
#1119=FACE_OUTER_BOUND('',#1516,.T.);
#1120=FACE_OUTER_BOUND('',#1517,.T.);
#1121=FACE_OUTER_BOUND('',#1518,.T.);
#1122=FACE_OUTER_BOUND('',#1519,.T.);
#1123=FACE_OUTER_BOUND('',#1520,.T.);
#1124=FACE_OUTER_BOUND('',#1521,.T.);
#1125=FACE_OUTER_BOUND('',#1522,.T.);
#1126=FACE_OUTER_BOUND('',#1523,.T.);
#1127=FACE_OUTER_BOUND('',#1524,.T.);
#1128=FACE_OUTER_BOUND('',#1525,.T.);
#1129=FACE_OUTER_BOUND('',#1526,.T.);
#1130=FACE_OUTER_BOUND('',#1527,.T.);
#1131=FACE_OUTER_BOUND('',#1528,.T.);
#1132=FACE_OUTER_BOUND('',#1529,.T.);
#1133=FACE_OUTER_BOUND('',#1532,.T.);
#1134=FACE_OUTER_BOUND('',#1533,.T.);
#1135=FACE_OUTER_BOUND('',#1534,.T.);
#1136=FACE_OUTER_BOUND('',#1535,.T.);
#1137=FACE_OUTER_BOUND('',#1536,.T.);
#1138=FACE_OUTER_BOUND('',#1537,.T.);
#1139=FACE_OUTER_BOUND('',#1538,.T.);
#1140=FACE_OUTER_BOUND('',#1539,.T.);
#1141=FACE_OUTER_BOUND('',#1540,.T.);
#1142=FACE_OUTER_BOUND('',#1541,.T.);
#1143=FACE_OUTER_BOUND('',#1542,.T.);
#1144=FACE_OUTER_BOUND('',#1543,.T.);
#1145=FACE_OUTER_BOUND('',#1544,.T.);
#1146=FACE_OUTER_BOUND('',#1545,.T.);
#1147=FACE_OUTER_BOUND('',#1546,.T.);
#1148=FACE_OUTER_BOUND('',#1547,.T.);
#1149=FACE_OUTER_BOUND('',#1548,.T.);
#1150=FACE_OUTER_BOUND('',#1549,.T.);
#1151=FACE_OUTER_BOUND('',#1550,.T.);
#1152=FACE_OUTER_BOUND('',#1551,.T.);
#1153=FACE_OUTER_BOUND('',#1552,.T.);
#1154=FACE_OUTER_BOUND('',#1553,.T.);
#1155=FACE_OUTER_BOUND('',#1554,.T.);
#1156=FACE_OUTER_BOUND('',#1555,.T.);
#1157=FACE_OUTER_BOUND('',#1556,.T.);
#1158=FACE_OUTER_BOUND('',#1558,.T.);
#1159=FACE_OUTER_BOUND('',#1559,.T.);
#1438=EDGE_LOOP('',(#4124,#4125,#4126,#4127,#4128,#4129));
#1439=EDGE_LOOP('',(#4130));
#1440=EDGE_LOOP('',(#4131,#4132,#4133,#4134,#4135));
#1441=EDGE_LOOP('',(#4136,#4137,#4138,#4139,#4140));
#1442=EDGE_LOOP('',(#4141));
#1443=EDGE_LOOP('',(#4142));
#1444=EDGE_LOOP('',(#4143,#4144,#4145,#4146));
#1445=EDGE_LOOP('',(#4147,#4148));
#1446=EDGE_LOOP('',(#4149));
#1447=EDGE_LOOP('',(#4150));
#1448=EDGE_LOOP('',(#4151,#4152,#4153,#4154,#4155));
#1449=EDGE_LOOP('',(#4156,#4157,#4158,#4159,#4160));
#1450=EDGE_LOOP('',(#4161,#4162,#4163,#4164,#4165,#4166));
#1451=EDGE_LOOP('',(#4167));
#1452=EDGE_LOOP('',(#4168,#4169,#4170,#4171));
#1453=EDGE_LOOP('',(#4172,#4173,#4174,#4175));
#1454=EDGE_LOOP('',(#4176,#4177,#4178,#4179));
#1455=EDGE_LOOP('',(#4180,#4181,#4182));
#1456=EDGE_LOOP('',(#4183,#4184,#4185,#4186));
#1457=EDGE_LOOP('',(#4187,#4188,#4189,#4190));
#1458=EDGE_LOOP('',(#4191,#4192,#4193,#4194));
#1459=EDGE_LOOP('',(#4195,#4196,#4197,#4198,#4199));
#1460=EDGE_LOOP('',(#4200,#4201,#4202,#4203));
#1461=EDGE_LOOP('',(#4204,#4205,#4206,#4207,#4208,#4209,#4210,#4211,#4212));
#1462=EDGE_LOOP('',(#4213,#4214,#4215,#4216));
#1463=EDGE_LOOP('',(#4217,#4218,#4219,#4220));
#1464=EDGE_LOOP('',(#4221,#4222,#4223));
#1465=EDGE_LOOP('',(#4224,#4225,#4226,#4227));
#1466=EDGE_LOOP('',(#4228,#4229,#4230));
#1467=EDGE_LOOP('',(#4231,#4232,#4233,#4234));
#1468=EDGE_LOOP('',(#4235,#4236,#4237));
#1469=EDGE_LOOP('',(#4238,#4239,#4240,#4241));
#1470=EDGE_LOOP('',(#4242,#4243,#4244,#4245));
#1471=EDGE_LOOP('',(#4246,#4247,#4248,#4249));
#1472=EDGE_LOOP('',(#4250,#4251,#4252));
#1473=EDGE_LOOP('',(#4253,#4254,#4255,#4256));
#1474=EDGE_LOOP('',(#4257,#4258,#4259));
#1475=EDGE_LOOP('',(#4260,#4261,#4262,#4263));
#1476=EDGE_LOOP('',(#4264,#4265,#4266,#4267));
#1477=EDGE_LOOP('',(#4268,#4269,#4270,#4271));
#1478=EDGE_LOOP('',(#4272));
#1479=EDGE_LOOP('',(#4273,#4274,#4275,#4276));
#1480=EDGE_LOOP('',(#4277,#4278,#4279));
#1481=EDGE_LOOP('',(#4280,#4281,#4282));
#1482=EDGE_LOOP('',(#4283,#4284,#4285,#4286));
#1483=EDGE_LOOP('',(#4287,#4288,#4289,#4290));
#1484=EDGE_LOOP('',(#4291));
#1485=EDGE_LOOP('',(#4292));
#1486=EDGE_LOOP('',(#4293,#4294,#4295,#4296));
#1487=EDGE_LOOP('',(#4297,#4298,#4299,#4300,#4301));
#1488=EDGE_LOOP('',(#4302,#4303,#4304,#4305,#4306,#4307));
#1489=EDGE_LOOP('',(#4308,#4309,#4310,#4311,#4312,#4313));
#1490=EDGE_LOOP('',(#4314,#4315,#4316,#4317,#4318,#4319));
#1491=EDGE_LOOP('',(#4320,#4321,#4322,#4323,#4324,#4325,#4326,#4327,#4328,
#4329,#4330,#4331,#4332,#4333));
#1492=EDGE_LOOP('',(#4334,#4335,#4336,#4337));
#1493=EDGE_LOOP('',(#4338,#4339,#4340,#4341,#4342,#4343,#4344,#4345,#4346,
#4347,#4348));
#1494=EDGE_LOOP('',(#4349));
#1495=EDGE_LOOP('',(#4350,#4351,#4352,#4353,#4354,#4355,#4356,#4357,#4358));
#1496=EDGE_LOOP('',(#4359));
#1497=EDGE_LOOP('',(#4360,#4361,#4362,#4363,#4364,#4365));
#1498=EDGE_LOOP('',(#4366,#4367,#4368,#4369,#4370,#4371,#4372,#4373,#4374));
#1499=EDGE_LOOP('',(#4375));
#1500=EDGE_LOOP('',(#4376,#4377,#4378,#4379,#4380,#4381,#4382,#4383,#4384,
#4385));
#1501=EDGE_LOOP('',(#4386));
#1502=EDGE_LOOP('',(#4387));
#1503=EDGE_LOOP('',(#4388,#4389,#4390,#4391,#4392,#4393,#4394));
#1504=EDGE_LOOP('',(#4395,#4396,#4397,#4398,#4399,#4400,#4401,#4402,#4403,
#4404));
#1505=EDGE_LOOP('',(#4405,#4406,#4407,#4408,#4409,#4410,#4411,#4412,#4413,
#4414,#4415,#4416));
#1506=EDGE_LOOP('',(#4417));
#1507=EDGE_LOOP('',(#4418));
#1508=EDGE_LOOP('',(#4419,#4420,#4421,#4422,#4423));
#1509=EDGE_LOOP('',(#4424,#4425,#4426,#4427));
#1510=EDGE_LOOP('',(#4428,#4429,#4430,#4431,#4432,#4433,#4434,#4435,#4436,
#4437,#4438,#4439));
#1511=EDGE_LOOP('',(#4440));
#1512=EDGE_LOOP('',(#4441,#4442,#4443,#4444));
#1513=EDGE_LOOP('',(#4445,#4446,#4447,#4448));
#1514=EDGE_LOOP('',(#4449,#4450,#4451,#4452));
#1515=EDGE_LOOP('',(#4453,#4454,#4455));
#1516=EDGE_LOOP('',(#4456,#4457,#4458));
#1517=EDGE_LOOP('',(#4459,#4460,#4461));
#1518=EDGE_LOOP('',(#4462,#4463,#4464));
#1519=EDGE_LOOP('',(#4465,#4466,#4467,#4468));
#1520=EDGE_LOOP('',(#4469,#4470,#4471,#4472));
#1521=EDGE_LOOP('',(#4473,#4474,#4475,#4476));
#1522=EDGE_LOOP('',(#4477,#4478,#4479,#4480));
#1523=EDGE_LOOP('',(#4481,#4482,#4483,#4484));
#1524=EDGE_LOOP('',(#4485,#4486,#4487,#4488));
#1525=EDGE_LOOP('',(#4489,#4490,#4491,#4492));
#1526=EDGE_LOOP('',(#4493,#4494,#4495,#4496,#4497));
#1527=EDGE_LOOP('',(#4498,#4499,#4500,#4501,#4502,#4503,#4504));
#1528=EDGE_LOOP('',(#4505,#4506,#4507,#4508,#4509));
#1529=EDGE_LOOP('',(#4510,#4511,#4512,#4513,#4514,#4515,#4516,#4517));
#1530=EDGE_LOOP('',(#4518));
#1531=EDGE_LOOP('',(#4519));
#1532=EDGE_LOOP('',(#4520,#4521,#4522,#4523));
#1533=EDGE_LOOP('',(#4524,#4525,#4526,#4527,#4528,#4529));
#1534=EDGE_LOOP('',(#4530,#4531,#4532,#4533));
#1535=EDGE_LOOP('',(#4534,#4535,#4536));
#1536=EDGE_LOOP('',(#4537,#4538,#4539,#4540));
#1537=EDGE_LOOP('',(#4541,#4542,#4543,#4544));
#1538=EDGE_LOOP('',(#4545,#4546,#4547,#4548));
#1539=EDGE_LOOP('',(#4549,#4550,#4551));
#1540=EDGE_LOOP('',(#4552,#4553,#4554,#4555));
#1541=EDGE_LOOP('',(#4556,#4557,#4558,#4559));
#1542=EDGE_LOOP('',(#4560,#4561,#4562,#4563));
#1543=EDGE_LOOP('',(#4564,#4565,#4566,#4567));
#1544=EDGE_LOOP('',(#4568,#4569,#4570,#4571));
#1545=EDGE_LOOP('',(#4572,#4573,#4574,#4575));
#1546=EDGE_LOOP('',(#4576,#4577,#4578));
#1547=EDGE_LOOP('',(#4579,#4580,#4581,#4582));
#1548=EDGE_LOOP('',(#4583,#4584,#4585,#4586));
#1549=EDGE_LOOP('',(#4587,#4588,#4589));
#1550=EDGE_LOOP('',(#4590,#4591,#4592,#4593));
#1551=EDGE_LOOP('',(#4594,#4595,#4596,#4597));
#1552=EDGE_LOOP('',(#4598,#4599,#4600,#4601));
#1553=EDGE_LOOP('',(#4602,#4603,#4604,#4605));
#1554=EDGE_LOOP('',(#4606,#4607,#4608,#4609));
#1555=EDGE_LOOP('',(#4610,#4611,#4612,#4613));
#1556=EDGE_LOOP('',(#4614));
#1557=EDGE_LOOP('',(#4615));
#1558=EDGE_LOOP('',(#4616,#4617,#4618,#4619));
#1559=EDGE_LOOP('',(#4620));
#1560=EDGE_LOOP('',(#4621));
#1924=LINE('',#9105,#2285);
#1925=LINE('',#9107,#2286);
#1926=LINE('',#9109,#2287);
#1927=LINE('',#9123,#2288);
#1928=LINE('',#9124,#2289);
#1929=LINE('',#9129,#2290);
#1930=LINE('',#9142,#2291);
#1931=LINE('',#9193,#2292);
#1932=LINE('',#9198,#2293);
#1933=LINE('',#9200,#2294);
#1934=LINE('',#9202,#2295);
#1935=LINE('',#9204,#2296);
#1936=LINE('',#9217,#2297);
#1937=LINE('',#9221,#2298);
#1938=LINE('',#9226,#2299);
#1939=LINE('',#9228,#2300);
#1940=LINE('',#9229,#2301);
#1941=LINE('',#9234,#2302);
#1942=LINE('',#9241,#2303);
#1943=LINE('',#9348,#2304);
#1944=LINE('',#9352,#2305);
#1945=LINE('',#9360,#2306);
#1946=LINE('',#9361,#2307);
#1947=LINE('',#9488,#2308);
#1948=LINE('',#9494,#2309);
#1949=LINE('',#9498,#2310);
#1950=LINE('',#9499,#2311);
#1951=LINE('',#9504,#2312);
#1952=LINE('',#9510,#2313);
#1953=LINE('',#9518,#2314);
#1954=LINE('',#9521,#2315);
#1955=LINE('',#9534,#2316);
#1956=LINE('',#9541,#2317);
#1957=LINE('',#9543,#2318);
#1958=LINE('',#9548,#2319);
#1959=LINE('',#9556,#2320);
#1960=LINE('',#9880,#2321);
#1961=LINE('',#9882,#2322);
#1962=LINE('',#9884,#2323);
#1963=LINE('',#9886,#2324);
#1964=LINE('',#9890,#2325);
#1965=LINE('',#9892,#2326);
#1966=LINE('',#9894,#2327);
#1967=LINE('',#9896,#2328);
#1968=LINE('',#9897,#2329);
#1969=LINE('',#9902,#2330);
#1970=LINE('',#9935,#2331);
#1971=LINE('',#9958,#2332);
#1972=LINE('',#9964,#2333);
#1973=LINE('',#9966,#2334);
#1974=LINE('',#9969,#2335);
#1975=LINE('',#9970,#2336);
#1976=LINE('',#9976,#2337);
#1977=LINE('',#9977,#2338);
#1978=LINE('',#9986,#2339);
#1979=LINE('',#9988,#2340);
#1980=LINE('',#9990,#2341);
#1981=LINE('',#9992,#2342);
#1982=LINE('',#9994,#2343);
#1983=LINE('',#10029,#2344);
#1984=LINE('',#10061,#2345);
#1985=LINE('',#10063,#2346);
#1986=LINE('',#10068,#2347);
#1987=LINE('',#10070,#2348);
#1988=LINE('',#10072,#2349);
#1989=LINE('',#10095,#2350);
#1990=LINE('',#10097,#2351);
#1991=LINE('',#10099,#2352);
#1992=LINE('',#10100,#2353);
#1993=LINE('',#10107,#2354);
#1994=LINE('',#10109,#2355);
#1995=LINE('',#10120,#2356);
#1996=LINE('',#10121,#2357);
#1997=LINE('',#10123,#2358);
#1998=LINE('',#10124,#2359);
#1999=LINE('',#10126,#2360);
#2000=LINE('',#10128,#2361);
#2001=LINE('',#10130,#2362);
#2002=LINE('',#10132,#2363);
#2003=LINE('',#10134,#2364);
#2004=LINE('',#10139,#2365);
#2005=LINE('',#10144,#2366);
#2006=LINE('',#10146,#2367);
#2007=LINE('',#10149,#2368);
#2008=LINE('',#10151,#2369);
#2009=LINE('',#10262,#2370);
#2010=LINE('',#10264,#2371);
#2011=LINE('',#10270,#2372);
#2012=LINE('',#10272,#2373);
#2013=LINE('',#10273,#2374);
#2014=LINE('',#10278,#2375);
#2015=LINE('',#10283,#2376);
#2016=LINE('',#10288,#2377);
#2017=LINE('',#10293,#2378);
#2018=LINE('',#10297,#2379);
#2019=LINE('',#10299,#2380);
#2020=LINE('',#10300,#2381);
#2021=LINE('',#10308,#2382);
#2022=LINE('',#10311,#2383);
#2023=LINE('',#10312,#2384);
#2024=LINE('',#10325,#2385);
#2025=LINE('',#10328,#2386);
#2026=LINE('',#10329,#2387);
#2027=LINE('',#10344,#2388);
#2028=LINE('',#10346,#2389);
#2029=LINE('',#10352,#2390);
#2030=LINE('',#10361,#2391);
#2285=VECTOR('',#7230,14.);
#2286=VECTOR('',#7231,14.);
#2287=VECTOR('',#7232,5.371378300226);
#2288=VECTOR('',#7233,5.371378300181);
#2289=VECTOR('',#7234,14.);
#2290=VECTOR('',#7239,4.5);
#2291=VECTOR('',#7256,2.5);
#2292=VECTOR('',#7273,4.5);
#2293=VECTOR('',#7278,14.);
#2294=VECTOR('',#7279,14.);
#2295=VECTOR('',#7280,14.);
#2296=VECTOR('',#7281,5.371378300226);
#2297=VECTOR('',#7282,5.371378300181);
#2298=VECTOR('',#7285,14.);
#2299=VECTOR('',#7292,12.);
#2300=VECTOR('',#7293,14.);
#2301=VECTOR('',#7294,12.);
#2302=VECTOR('',#7299,12.);
#2303=VECTOR('',#7310,5.371378297288);
#2304=VECTOR('',#7317,5.371378302463);
#2305=VECTOR('',#7322,5.371378302463);
#2306=VECTOR('',#7331,5.371378297288);
#2307=VECTOR('',#7332,12.);
#2308=VECTOR('',#7363,12.);
#2309=VECTOR('',#7372,14.);
#2310=VECTOR('',#7377,14.);
#2311=VECTOR('',#7378,12.);
#2312=VECTOR('',#7383,12.);
#2313=VECTOR('',#7392,14.);
#2314=VECTOR('',#7405,12.);
#2315=VECTOR('',#7410,14.);
#2316=VECTOR('',#7431,4.);
#2317=VECTOR('',#7440,1.375);
#2318=VECTOR('',#7443,1.25);
#2319=VECTOR('',#7448,5.187242561534);
#2320=VECTOR('',#7457,5.187242561534);
#2321=VECTOR('',#7484,2.868878241544);
#2322=VECTOR('',#7485,1.868875965277);
#2323=VECTOR('',#7486,30.);
#2324=VECTOR('',#7487,14.);
#2325=VECTOR('',#7490,14.26794919243);
#2326=VECTOR('',#7491,1.);
#2327=VECTOR('',#7492,7.);
#2328=VECTOR('',#7493,1.);
#2329=VECTOR('',#7494,9.);
#2330=VECTOR('',#7499,2.625);
#2331=VECTOR('',#7500,2.625);
#2332=VECTOR('',#7507,1.75);
#2333=VECTOR('',#7514,24.);
#2334=VECTOR('',#7515,9.);
#2335=VECTOR('',#7518,10.);
#2336=VECTOR('',#7519,10.);
#2337=VECTOR('',#7524,14.26794919243);
#2338=VECTOR('',#7525,24.);
#2339=VECTOR('',#7526,7.);
#2340=VECTOR('',#7527,4.);
#2341=VECTOR('',#7528,40.);
#2342=VECTOR('',#7529,4.);
#2343=VECTOR('',#7530,7.);
#2344=VECTOR('',#7535,1.75);
#2345=VECTOR('',#7540,2.625);
#2346=VECTOR('',#7541,2.625);
#2347=VECTOR('',#7546,14.);
#2348=VECTOR('',#7547,30.);
#2349=VECTOR('',#7548,1.868878442791);
#2350=VECTOR('',#7549,2.868877901305);
#2351=VECTOR('',#7550,1.);
#2352=VECTOR('',#7551,7.);
#2353=VECTOR('',#7552,1.);
#2354=VECTOR('',#7561,7.);
#2355=VECTOR('',#7562,7.);
#2356=VECTOR('',#7575,31.);
#2357=VECTOR('',#7576,10.);
#2358=VECTOR('',#7577,10.);
#2359=VECTOR('',#7578,31.);
#2360=VECTOR('',#7579,7.);
#2361=VECTOR('',#7580,4.);
#2362=VECTOR('',#7581,40.);
#2363=VECTOR('',#7582,4.);
#2364=VECTOR('',#7583,7.);
#2365=VECTOR('',#7590,2.);
#2366=VECTOR('',#7599,2.868880399918);
#2367=VECTOR('',#7602,2.868878955581);
#2368=VECTOR('',#7607,2.868878761621);
#2369=VECTOR('',#7610,2.868878597225);
#2370=VECTOR('',#7635,7.);
#2371=VECTOR('',#7636,7.);
#2372=VECTOR('',#7643,7.);
#2373=VECTOR('',#7644,14.);
#2374=VECTOR('',#7645,7.);
#2375=VECTOR('',#7652,2.);
#2376=VECTOR('',#7657,14.);
#2377=VECTOR('',#7662,14.);
#2378=VECTOR('',#7669,2.);
#2379=VECTOR('',#7674,7.);
#2380=VECTOR('',#7675,14.);
#2381=VECTOR('',#7676,7.);
#2382=VECTOR('',#7689,4.);
#2383=VECTOR('',#7692,4.);
#2384=VECTOR('',#7693,14.);
#2385=VECTOR('',#7716,4.);
#2386=VECTOR('',#7719,14.);
#2387=VECTOR('',#7720,4.);
#2388=VECTOR('',#7749,24.);
#2389=VECTOR('',#7752,24.);
#2390=VECTOR('',#7759,3.);
#2391=VECTOR('',#7770,3.);
#2650=VERTEX_POINT('',#9103);
#2651=VERTEX_POINT('',#9104);
#2652=VERTEX_POINT('',#9106);
#2653=VERTEX_POINT('',#9108);
#2654=VERTEX_POINT('',#9110);
#2655=VERTEX_POINT('',#9122);
#2656=VERTEX_POINT('',#9125);
#2657=VERTEX_POINT('',#9128);
#2658=VERTEX_POINT('',#9130);
#2659=VERTEX_POINT('',#9134);
#2660=VERTEX_POINT('',#9138);
#2661=VERTEX_POINT('',#9141);
#2662=VERTEX_POINT('',#9144);
#2663=VERTEX_POINT('',#9145);
#2664=VERTEX_POINT('',#9183);
#2665=VERTEX_POINT('',#9186);
#2666=VERTEX_POINT('',#9188);
#2667=VERTEX_POINT('',#9192);
#2668=VERTEX_POINT('',#9196);
#2669=VERTEX_POINT('',#9197);
#2670=VERTEX_POINT('',#9199);
#2671=VERTEX_POINT('',#9201);
#2672=VERTEX_POINT('',#9203);
#2673=VERTEX_POINT('',#9205);
#2674=VERTEX_POINT('',#9219);
#2675=VERTEX_POINT('',#9220);
#2676=VERTEX_POINT('',#9225);
#2677=VERTEX_POINT('',#9227);
#2678=VERTEX_POINT('',#9231);
#2679=VERTEX_POINT('',#9233);
#2680=VERTEX_POINT('',#9240);
#2681=VERTEX_POINT('',#9295);
#2682=VERTEX_POINT('',#9347);
#2683=VERTEX_POINT('',#9351);
#2684=VERTEX_POINT('',#9353);
#2685=VERTEX_POINT('',#9357);
#2686=VERTEX_POINT('',#9359);
#2687=VERTEX_POINT('',#9363);
#2688=VERTEX_POINT('',#9365);
#2689=VERTEX_POINT('',#9483);
#2690=VERTEX_POINT('',#9487);
#2691=VERTEX_POINT('',#9493);
#2692=VERTEX_POINT('',#9497);
#2693=VERTEX_POINT('',#9501);
#2694=VERTEX_POINT('',#9503);
#2695=VERTEX_POINT('',#9509);
#2696=VERTEX_POINT('',#9517);
#2697=VERTEX_POINT('',#9522);
#2698=VERTEX_POINT('',#9532);
#2699=VERTEX_POINT('',#9536);
#2700=VERTEX_POINT('',#9539);
#2701=VERTEX_POINT('',#9545);
#2702=VERTEX_POINT('',#9546);
#2703=VERTEX_POINT('',#9551);
#2704=VERTEX_POINT('',#9552);
#2705=VERTEX_POINT('',#9555);
#2706=VERTEX_POINT('',#9557);
#2707=VERTEX_POINT('',#9563);
#2708=VERTEX_POINT('',#9565);
#2709=VERTEX_POINT('',#9576);
#2710=VERTEX_POINT('',#9578);
#2711=VERTEX_POINT('',#9622);
#2712=VERTEX_POINT('',#9669);
#2713=VERTEX_POINT('',#9671);
#2714=VERTEX_POINT('',#9691);
#2715=VERTEX_POINT('',#9693);
#2716=VERTEX_POINT('',#9776);
#2717=VERTEX_POINT('',#9859);
#2718=VERTEX_POINT('',#9860);
#2719=VERTEX_POINT('',#9879);
#2720=VERTEX_POINT('',#9881);
#2721=VERTEX_POINT('',#9883);
#2722=VERTEX_POINT('',#9885);
#2723=VERTEX_POINT('',#9887);
#2724=VERTEX_POINT('',#9889);
#2725=VERTEX_POINT('',#9891);
#2726=VERTEX_POINT('',#9893);
#2727=VERTEX_POINT('',#9895);
#2728=VERTEX_POINT('',#9898);
#2729=VERTEX_POINT('',#9901);
#2730=VERTEX_POINT('',#9903);
#2731=VERTEX_POINT('',#9908);
#2732=VERTEX_POINT('',#9934);
#2733=VERTEX_POINT('',#9957);
#2734=VERTEX_POINT('',#9961);
#2735=VERTEX_POINT('',#9963);
#2736=VERTEX_POINT('',#9965);
#2737=VERTEX_POINT('',#9967);
#2738=VERTEX_POINT('',#9971);
#2739=VERTEX_POINT('',#9974);
#2740=VERTEX_POINT('',#9975);
#2741=VERTEX_POINT('',#9978);
#2742=VERTEX_POINT('',#9985);
#2743=VERTEX_POINT('',#9987);
#2744=VERTEX_POINT('',#9989);
#2745=VERTEX_POINT('',#9991);
#2746=VERTEX_POINT('',#9993);
#2747=VERTEX_POINT('',#10001);
#2748=VERTEX_POINT('',#10004);
#2749=VERTEX_POINT('',#10005);
#2750=VERTEX_POINT('',#10030);
#2751=VERTEX_POINT('',#10035);
#2752=VERTEX_POINT('',#10059);
#2753=VERTEX_POINT('',#10062);
#2754=VERTEX_POINT('',#10066);
#2755=VERTEX_POINT('',#10067);
#2756=VERTEX_POINT('',#10069);
#2757=VERTEX_POINT('',#10071);
#2758=VERTEX_POINT('',#10073);
#2759=VERTEX_POINT('',#10085);
#2760=VERTEX_POINT('',#10096);
#2761=VERTEX_POINT('',#10098);
#2762=VERTEX_POINT('',#10104);
#2763=VERTEX_POINT('',#10106);
#2764=VERTEX_POINT('',#10108);
#2765=VERTEX_POINT('',#10112);
#2766=VERTEX_POINT('',#10113);
#2767=VERTEX_POINT('',#10118);
#2768=VERTEX_POINT('',#10119);
#2769=VERTEX_POINT('',#10122);
#2770=VERTEX_POINT('',#10125);
#2771=VERTEX_POINT('',#10127);
#2772=VERTEX_POINT('',#10129);
#2773=VERTEX_POINT('',#10131);
#2774=VERTEX_POINT('',#10133);
#2775=VERTEX_POINT('',#10136);
#2776=VERTEX_POINT('',#10257);
#2777=VERTEX_POINT('',#10261);
#2778=VERTEX_POINT('',#10263);
#2779=VERTEX_POINT('',#10267);
#2780=VERTEX_POINT('',#10269);
#2781=VERTEX_POINT('',#10271);
#2782=VERTEX_POINT('',#10276);
#2783=VERTEX_POINT('',#10280);
#2784=VERTEX_POINT('',#10282);
#2785=VERTEX_POINT('',#10285);
#2786=VERTEX_POINT('',#10287);
#2787=VERTEX_POINT('',#10290);
#2788=VERTEX_POINT('',#10296);
#2789=VERTEX_POINT('',#10298);
#2790=VERTEX_POINT('',#10304);
#2791=VERTEX_POINT('',#10310);
#2792=VERTEX_POINT('',#10323);
#2793=VERTEX_POINT('',#10327);
#2794=VERTEX_POINT('',#10349);
#2795=VERTEX_POINT('',#10351);
#2796=VERTEX_POINT('',#10355);
#2797=VERTEX_POINT('',#10358);
#2798=VERTEX_POINT('',#10360);
#2799=VERTEX_POINT('',#10364);
#3210=EDGE_CURVE('',#2650,#2651,#1924,.T.);
#3211=EDGE_CURVE('',#2651,#2652,#1925,.T.);
#3212=EDGE_CURVE('',#2652,#2653,#1926,.T.);
#3213=EDGE_CURVE('',#2653,#2654,#146,.T.);
#3214=EDGE_CURVE('',#2654,#2655,#1927,.T.);
#3215=EDGE_CURVE('',#2655,#2650,#1928,.T.);
#3216=EDGE_CURVE('',#2656,#2656,#678,.T.);
#3217=EDGE_CURVE('',#2656,#2657,#1929,.T.);
#3218=EDGE_CURVE('',#2658,#2657,#679,.T.);
#3219=EDGE_CURVE('',#2657,#2658,#680,.T.);
#3220=EDGE_CURVE('',#2658,#2659,#681,.T.);
#3221=EDGE_CURVE('',#2659,#2659,#682,.T.);
#3222=EDGE_CURVE('',#2660,#2660,#683,.T.);
#3223=EDGE_CURVE('',#2660,#2661,#1930,.T.);
#3224=EDGE_CURVE('',#2661,#2661,#684,.T.);
#3225=EDGE_CURVE('',#2662,#2663,#147,.T.);
#3226=EDGE_CURVE('',#2663,#2662,#148,.T.);
#3227=EDGE_CURVE('',#2664,#2664,#685,.T.);
#3228=EDGE_CURVE('',#2664,#2665,#686,.T.);
#3229=EDGE_CURVE('',#2665,#2666,#687,.T.);
#3230=EDGE_CURVE('',#2666,#2665,#688,.T.);
#3231=EDGE_CURVE('',#2666,#2667,#1931,.T.);
#3232=EDGE_CURVE('',#2667,#2667,#689,.T.);
#3233=EDGE_CURVE('',#2668,#2669,#1932,.T.);
#3234=EDGE_CURVE('',#2669,#2670,#1933,.T.);
#3235=EDGE_CURVE('',#2670,#2671,#1934,.T.);
#3236=EDGE_CURVE('',#2671,#2672,#1935,.T.);
#3237=EDGE_CURVE('',#2672,#2673,#149,.T.);
#3238=EDGE_CURVE('',#2673,#2668,#1936,.T.);
#3239=EDGE_CURVE('',#2674,#2675,#1937,.T.);
#3240=EDGE_CURVE('',#2669,#2675,#690,.T.);
#3241=EDGE_CURVE('',#2674,#2668,#691,.T.);
#3242=EDGE_CURVE('',#2674,#2676,#1938,.T.);
#3243=EDGE_CURVE('',#2677,#2676,#1939,.T.);
#3244=EDGE_CURVE('',#2675,#2677,#1940,.T.);
#3245=EDGE_CURVE('',#2678,#2674,#692,.T.);
#3246=EDGE_CURVE('',#2678,#2679,#1941,.T.);
#3247=EDGE_CURVE('',#2676,#2679,#693,.T.);
#3248=EDGE_CURVE('',#2679,#2652,#694,.T.);
#3249=EDGE_CURVE('',#2652,#2676,#695,.T.);
#3250=EDGE_CURVE('',#2679,#2680,#1942,.T.);
#3251=EDGE_CURVE('',#2653,#2680,#696,.T.);
#3252=EDGE_CURVE('',#2680,#2681,#150,.T.);
#3253=EDGE_CURVE('',#2654,#2681,#697,.T.);
#3254=EDGE_CURVE('',#2681,#2682,#1943,.T.);
#3255=EDGE_CURVE('',#2655,#2682,#698,.T.);
#3256=EDGE_CURVE('',#2683,#2678,#1944,.T.);
#3257=EDGE_CURVE('',#2684,#2683,#699,.T.);
#3258=EDGE_CURVE('',#2680,#2684,#700,.T.);
#3259=EDGE_CURVE('',#2685,#2681,#701,.T.);
#3260=EDGE_CURVE('',#2686,#2685,#1945,.T.);
#3261=EDGE_CURVE('',#2686,#2682,#1946,.T.);
#3262=EDGE_CURVE('',#2684,#2687,#702,.T.);
#3263=EDGE_CURVE('',#2688,#2687,#703,.T.);
#3264=EDGE_CURVE('',#2687,#2688,#704,.T.);
#3265=EDGE_CURVE('',#2685,#2683,#151,.T.);
#3266=EDGE_CURVE('',#2672,#2685,#705,.T.);
#3267=EDGE_CURVE('',#2673,#2683,#706,.T.);
#3268=EDGE_CURVE('',#2668,#2678,#707,.T.);
#3269=EDGE_CURVE('',#2686,#2671,#708,.T.);
#3270=EDGE_CURVE('',#2671,#2689,#709,.T.);
#3271=EDGE_CURVE('',#2689,#2686,#710,.T.);
#3272=EDGE_CURVE('',#2689,#2690,#1947,.T.);
#3273=EDGE_CURVE('',#2682,#2690,#711,.T.);
#3274=EDGE_CURVE('',#2690,#2655,#712,.T.);
#3275=EDGE_CURVE('',#2690,#2691,#1948,.T.);
#3276=EDGE_CURVE('',#2650,#2691,#713,.T.);
#3277=EDGE_CURVE('',#2692,#2689,#1949,.T.);
#3278=EDGE_CURVE('',#2692,#2691,#1950,.T.);
#3279=EDGE_CURVE('',#2693,#2692,#714,.T.);
#3280=EDGE_CURVE('',#2693,#2694,#1951,.T.);
#3281=EDGE_CURVE('',#2691,#2694,#715,.T.);
#3282=EDGE_CURVE('',#2694,#2650,#716,.T.);
#3283=EDGE_CURVE('',#2694,#2695,#1952,.T.);
#3284=EDGE_CURVE('',#2651,#2695,#717,.T.);
#3285=EDGE_CURVE('',#2677,#2651,#718,.T.);
#3286=EDGE_CURVE('',#2695,#2677,#719,.T.);
#3287=EDGE_CURVE('',#2696,#2695,#1953,.T.);
#3288=EDGE_CURVE('',#2675,#2696,#720,.T.);
#3289=EDGE_CURVE('',#2696,#2693,#1954,.T.);
#3290=EDGE_CURVE('',#2697,#2697,#721,.T.);
#3291=EDGE_CURVE('',#2670,#2693,#722,.T.);
#3292=EDGE_CURVE('',#2696,#2669,#723,.T.);
#3293=EDGE_CURVE('',#2692,#2670,#724,.T.);
#3294=EDGE_CURVE('',#2698,#2698,#725,.T.);
#3295=EDGE_CURVE('',#2698,#2697,#1955,.T.);
#3296=EDGE_CURVE('',#2699,#2699,#726,.T.);
#3297=EDGE_CURVE('',#2700,#2700,#727,.T.);
#3298=EDGE_CURVE('',#2700,#2699,#1956,.T.);
#3299=EDGE_CURVE('',#2663,#2700,#1957,.T.);
#3300=EDGE_CURVE('',#2701,#2702,#728,.T.);
#3301=EDGE_CURVE('',#2702,#2688,#1958,.T.);
#3302=EDGE_CURVE('',#2702,#2701,#729,.T.);
#3303=EDGE_CURVE('',#2703,#2704,#730,.T.);
#3304=EDGE_CURVE('',#2704,#2703,#731,.T.);
#3305=EDGE_CURVE('',#2703,#2705,#1959,.T.);
#3306=EDGE_CURVE('',#2706,#2705,#732,.T.);
#3307=EDGE_CURVE('',#2705,#2706,#733,.T.);
#3308=EDGE_CURVE('',#2701,#2706,#734,.T.);
#3309=EDGE_CURVE('',#2704,#2707,#735,.T.);
#3310=EDGE_CURVE('',#2708,#2707,#152,.T.);
#3311=EDGE_CURVE('',#2708,#2709,#736,.T.);
#3312=EDGE_CURVE('',#2709,#2710,#153,.T.);
#3313=EDGE_CURVE('',#2710,#2711,#154,.T.);
#3314=EDGE_CURVE('',#2711,#2712,#737,.T.);
#3315=EDGE_CURVE('',#2712,#2713,#155,.F.);
#3316=EDGE_CURVE('',#2713,#2714,#738,.T.);
#3317=EDGE_CURVE('',#2715,#2714,#156,.T.);
#3318=EDGE_CURVE('',#2715,#2716,#739,.T.);
#3319=EDGE_CURVE('',#2707,#2716,#157,.T.);
#3320=EDGE_CURVE('',#2717,#2718,#158,.T.);
#3321=EDGE_CURVE('',#2717,#2715,#740,.T.);
#3322=EDGE_CURVE('',#2718,#2714,#741,.T.);
#3323=EDGE_CURVE('',#2719,#2717,#1960,.T.);
#3324=EDGE_CURVE('',#2718,#2720,#1961,.T.);
#3325=EDGE_CURVE('',#2721,#2720,#1962,.T.);
#3326=EDGE_CURVE('',#2721,#2722,#1963,.T.);
#3327=EDGE_CURVE('',#2722,#2723,#742,.T.);
#3328=EDGE_CURVE('',#2724,#2723,#1964,.T.);
#3329=EDGE_CURVE('',#2724,#2725,#1965,.T.);
#3330=EDGE_CURVE('',#2725,#2726,#1966,.T.);
#3331=EDGE_CURVE('',#2727,#2726,#1967,.T.);
#3332=EDGE_CURVE('',#2719,#2727,#1968,.T.);
#3333=EDGE_CURVE('',#2728,#2728,#743,.T.);
#3334=EDGE_CURVE('',#2728,#2729,#1969,.T.);
#3335=EDGE_CURVE('',#2730,#2729,#159,.F.);
#3336=EDGE_CURVE('',#2731,#2730,#160,.F.);
#3337=EDGE_CURVE('',#2731,#2732,#1970,.T.);
#3338=EDGE_CURVE('',#2732,#2732,#744,.T.);
#3339=EDGE_CURVE('',#2729,#2731,#161,.F.);
#3340=EDGE_CURVE('',#2730,#2733,#1971,.T.);
#3341=EDGE_CURVE('',#2733,#2733,#745,.T.);
#3342=EDGE_CURVE('',#2734,#2719,#746,.T.);
#3343=EDGE_CURVE('',#2727,#2735,#1972,.T.);
#3344=EDGE_CURVE('',#2735,#2736,#1973,.T.);
#3345=EDGE_CURVE('',#2736,#2737,#747,.T.);
#3346=EDGE_CURVE('',#2737,#2708,#1974,.T.);
#3347=EDGE_CURVE('',#2716,#2734,#1975,.T.);
#3348=EDGE_CURVE('',#2738,#2738,#748,.T.);
#3349=EDGE_CURVE('',#2739,#2740,#1976,.T.);
#3350=EDGE_CURVE('',#2724,#2740,#1977,.T.);
#3351=EDGE_CURVE('',#2741,#2723,#162,.T.);
#3352=EDGE_CURVE('',#2741,#2742,#1978,.T.);
#3353=EDGE_CURVE('',#2742,#2743,#1979,.T.);
#3354=EDGE_CURVE('',#2743,#2744,#1980,.T.);
#3355=EDGE_CURVE('',#2744,#2745,#1981,.T.);
#3356=EDGE_CURVE('',#2745,#2746,#1982,.T.);
#3357=EDGE_CURVE('',#2739,#2746,#163,.T.);
#3358=EDGE_CURVE('',#2747,#2747,#749,.T.);
#3359=EDGE_CURVE('',#2748,#2749,#164,.T.);
#3360=EDGE_CURVE('',#2749,#2747,#1983,.T.);
#3361=EDGE_CURVE('',#2749,#2750,#165,.T.);
#3362=EDGE_CURVE('',#2750,#2751,#166,.T.);
#3363=EDGE_CURVE('',#2751,#2748,#167,.T.);
#3364=EDGE_CURVE('',#2752,#2752,#750,.T.);
#3365=EDGE_CURVE('',#2752,#2750,#1984,.T.);
#3366=EDGE_CURVE('',#2751,#2753,#1985,.T.);
#3367=EDGE_CURVE('',#2753,#2753,#751,.T.);
#3368=EDGE_CURVE('',#2754,#2755,#1986,.T.);
#3369=EDGE_CURVE('',#2756,#2754,#1987,.T.);
#3370=EDGE_CURVE('',#2757,#2756,#1988,.T.);
#3371=EDGE_CURVE('',#2758,#2757,#168,.T.);
#3372=EDGE_CURVE('',#2759,#2758,#169,.T.);
#3373=EDGE_CURVE('',#2736,#2759,#1989,.T.);
#3374=EDGE_CURVE('',#2735,#2760,#1990,.T.);
#3375=EDGE_CURVE('',#2761,#2760,#1991,.T.);
#3376=EDGE_CURVE('',#2740,#2761,#1992,.T.);
#3377=EDGE_CURVE('',#2739,#2755,#752,.T.);
#3378=EDGE_CURVE('',#2762,#2755,#753,.T.);
#3379=EDGE_CURVE('',#2763,#2762,#1993,.T.);
#3380=EDGE_CURVE('',#2764,#2763,#1994,.T.);
#3381=EDGE_CURVE('',#2754,#2764,#754,.T.);
#3382=EDGE_CURVE('',#2765,#2766,#755,.T.);
#3383=EDGE_CURVE('',#2765,#2754,#756,.T.);
#3384=EDGE_CURVE('',#2764,#2766,#757,.T.);
#3385=EDGE_CURVE('',#2767,#2768,#1995,.T.);
#3386=EDGE_CURVE('',#2713,#2768,#1996,.T.);
#3387=EDGE_CURVE('',#2769,#2712,#1997,.T.);
#3388=EDGE_CURVE('',#2769,#2765,#1998,.T.);
#3389=EDGE_CURVE('',#2766,#2770,#1999,.T.);
#3390=EDGE_CURVE('',#2770,#2771,#2000,.T.);
#3391=EDGE_CURVE('',#2772,#2771,#2001,.T.);
#3392=EDGE_CURVE('',#2772,#2773,#2002,.T.);
#3393=EDGE_CURVE('',#2773,#2774,#2003,.T.);
#3394=EDGE_CURVE('',#2774,#2767,#758,.T.);
#3395=EDGE_CURVE('',#2775,#2775,#759,.T.);
#3396=EDGE_CURVE('',#2775,#2738,#2004,.T.);
#3397=EDGE_CURVE('',#2721,#2767,#760,.T.);
#3398=EDGE_CURVE('',#2720,#2768,#105,.T.);
#3399=EDGE_CURVE('',#2714,#2768,#2005,.T.);
#3400=EDGE_CURVE('',#2734,#2715,#2006,.T.);
#3401=EDGE_CURVE('',#2737,#2709,#2007,.T.);
#3402=EDGE_CURVE('',#2711,#2769,#2008,.T.);
#3403=EDGE_CURVE('',#2709,#2759,#761,.T.);
#3404=EDGE_CURVE('',#2710,#2758,#762,.T.);
#3405=EDGE_CURVE('',#2711,#2757,#763,.T.);
#3406=EDGE_CURVE('',#2756,#2769,#106,.T.);
#3407=EDGE_CURVE('',#2774,#2776,#764,.T.);
#3408=EDGE_CURVE('',#2776,#2721,#765,.T.);
#3409=EDGE_CURVE('',#2776,#2777,#2009,.T.);
#3410=EDGE_CURVE('',#2777,#2778,#2010,.T.);
#3411=EDGE_CURVE('',#2722,#2778,#766,.T.);
#3412=EDGE_CURVE('',#2777,#2779,#767,.T.);
#3413=EDGE_CURVE('',#2780,#2776,#2011,.T.);
#3414=EDGE_CURVE('',#2781,#2780,#2012,.T.);
#3415=EDGE_CURVE('',#2778,#2781,#2013,.T.);
#3416=EDGE_CURVE('',#2779,#2777,#768,.T.);
#3417=EDGE_CURVE('',#2782,#2782,#769,.T.);
#3418=EDGE_CURVE('',#2782,#2779,#2014,.T.);
#3419=EDGE_CURVE('',#2743,#2783,#770,.T.);
#3420=EDGE_CURVE('',#2784,#2783,#2015,.T.);
#3421=EDGE_CURVE('',#2784,#2772,#771,.T.);
#3422=EDGE_CURVE('',#2771,#2785,#772,.T.);
#3423=EDGE_CURVE('',#2785,#2786,#2016,.T.);
#3424=EDGE_CURVE('',#2786,#2744,#773,.T.);
#3425=EDGE_CURVE('',#2787,#2787,#774,.T.);
#3426=EDGE_CURVE('',#2787,#2763,#2017,.T.);
#3427=EDGE_CURVE('',#2763,#2763,#775,.T.);
#3428=EDGE_CURVE('',#2788,#2762,#2018,.T.);
#3429=EDGE_CURVE('',#2788,#2789,#2019,.T.);
#3430=EDGE_CURVE('',#2764,#2789,#2020,.T.);
#3431=EDGE_CURVE('',#2770,#2789,#776,.T.);
#3432=EDGE_CURVE('',#2790,#2770,#777,.T.);
#3433=EDGE_CURVE('',#2789,#2790,#778,.T.);
#3434=EDGE_CURVE('',#2790,#2785,#2021,.T.);
#3435=EDGE_CURVE('',#2786,#2791,#2022,.T.);
#3436=EDGE_CURVE('',#2791,#2790,#2023,.T.);
#3437=EDGE_CURVE('',#2745,#2791,#779,.T.);
#3438=EDGE_CURVE('',#2788,#2745,#780,.T.);
#3439=EDGE_CURVE('',#2791,#2788,#781,.T.);
#3440=EDGE_CURVE('',#2746,#2762,#782,.T.);
#3441=EDGE_CURVE('',#2792,#2742,#783,.T.);
#3442=EDGE_CURVE('',#2792,#2783,#2024,.T.);
#3443=EDGE_CURVE('',#2792,#2793,#2025,.T.);
#3444=EDGE_CURVE('',#2784,#2793,#2026,.T.);
#3445=EDGE_CURVE('',#2773,#2793,#784,.T.);
#3446=EDGE_CURVE('',#2793,#2780,#785,.T.);
#3447=EDGE_CURVE('',#2780,#2773,#786,.T.);
#3448=EDGE_CURVE('',#2781,#2792,#787,.T.);
#3449=EDGE_CURVE('',#2742,#2781,#788,.T.);
#3450=EDGE_CURVE('',#2778,#2741,#789,.T.);
#3451=EDGE_CURVE('',#2725,#2761,#2027,.T.);
#3452=EDGE_CURVE('',#2726,#2760,#2028,.T.);
#3453=EDGE_CURVE('',#2794,#2794,#790,.T.);
#3454=EDGE_CURVE('',#2794,#2795,#2029,.T.);
#3455=EDGE_CURVE('',#2795,#2795,#791,.T.);
#3456=EDGE_CURVE('',#2796,#2796,#792,.T.);
#3457=EDGE_CURVE('',#2797,#2797,#793,.T.);
#3458=EDGE_CURVE('',#2797,#2798,#2030,.T.);
#3459=EDGE_CURVE('',#2798,#2798,#794,.T.);
#3460=EDGE_CURVE('',#2799,#2799,#795,.T.);
#4124=ORIENTED_EDGE('',*,*,#3210,.T.);
#4125=ORIENTED_EDGE('',*,*,#3211,.T.);
#4126=ORIENTED_EDGE('',*,*,#3212,.T.);
#4127=ORIENTED_EDGE('',*,*,#3213,.T.);
#4128=ORIENTED_EDGE('',*,*,#3214,.T.);
#4129=ORIENTED_EDGE('',*,*,#3215,.T.);
#4130=ORIENTED_EDGE('',*,*,#3216,.T.);
#4131=ORIENTED_EDGE('',*,*,#3216,.F.);
#4132=ORIENTED_EDGE('',*,*,#3217,.T.);
#4133=ORIENTED_EDGE('',*,*,#3218,.F.);
#4134=ORIENTED_EDGE('',*,*,#3219,.F.);
#4135=ORIENTED_EDGE('',*,*,#3217,.F.);
#4136=ORIENTED_EDGE('',*,*,#3218,.T.);
#4137=ORIENTED_EDGE('',*,*,#3219,.T.);
#4138=ORIENTED_EDGE('',*,*,#3220,.T.);
#4139=ORIENTED_EDGE('',*,*,#3221,.F.);
#4140=ORIENTED_EDGE('',*,*,#3220,.F.);
#4141=ORIENTED_EDGE('',*,*,#3221,.T.);
#4142=ORIENTED_EDGE('',*,*,#3222,.T.);
#4143=ORIENTED_EDGE('',*,*,#3222,.F.);
#4144=ORIENTED_EDGE('',*,*,#3223,.T.);
#4145=ORIENTED_EDGE('',*,*,#3224,.T.);
#4146=ORIENTED_EDGE('',*,*,#3223,.F.);
#4147=ORIENTED_EDGE('',*,*,#3225,.T.);
#4148=ORIENTED_EDGE('',*,*,#3226,.T.);
#4149=ORIENTED_EDGE('',*,*,#3227,.T.);
#4150=ORIENTED_EDGE('',*,*,#3224,.F.);
#4151=ORIENTED_EDGE('',*,*,#3227,.F.);
#4152=ORIENTED_EDGE('',*,*,#3228,.T.);
#4153=ORIENTED_EDGE('',*,*,#3229,.T.);
#4154=ORIENTED_EDGE('',*,*,#3230,.T.);
#4155=ORIENTED_EDGE('',*,*,#3228,.F.);
#4156=ORIENTED_EDGE('',*,*,#3229,.F.);
#4157=ORIENTED_EDGE('',*,*,#3230,.F.);
#4158=ORIENTED_EDGE('',*,*,#3231,.T.);
#4159=ORIENTED_EDGE('',*,*,#3232,.T.);
#4160=ORIENTED_EDGE('',*,*,#3231,.F.);
#4161=ORIENTED_EDGE('',*,*,#3233,.T.);
#4162=ORIENTED_EDGE('',*,*,#3234,.T.);
#4163=ORIENTED_EDGE('',*,*,#3235,.T.);
#4164=ORIENTED_EDGE('',*,*,#3236,.T.);
#4165=ORIENTED_EDGE('',*,*,#3237,.T.);
#4166=ORIENTED_EDGE('',*,*,#3238,.T.);
#4167=ORIENTED_EDGE('',*,*,#3232,.F.);
#4168=ORIENTED_EDGE('',*,*,#3239,.T.);
#4169=ORIENTED_EDGE('',*,*,#3240,.F.);
#4170=ORIENTED_EDGE('',*,*,#3233,.F.);
#4171=ORIENTED_EDGE('',*,*,#3241,.F.);
#4172=ORIENTED_EDGE('',*,*,#3242,.T.);
#4173=ORIENTED_EDGE('',*,*,#3243,.F.);
#4174=ORIENTED_EDGE('',*,*,#3244,.F.);
#4175=ORIENTED_EDGE('',*,*,#3239,.F.);
#4176=ORIENTED_EDGE('',*,*,#3242,.F.);
#4177=ORIENTED_EDGE('',*,*,#3245,.F.);
#4178=ORIENTED_EDGE('',*,*,#3246,.T.);
#4179=ORIENTED_EDGE('',*,*,#3247,.F.);
#4180=ORIENTED_EDGE('',*,*,#3248,.T.);
#4181=ORIENTED_EDGE('',*,*,#3249,.T.);
#4182=ORIENTED_EDGE('',*,*,#3247,.T.);
#4183=ORIENTED_EDGE('',*,*,#3212,.F.);
#4184=ORIENTED_EDGE('',*,*,#3248,.F.);
#4185=ORIENTED_EDGE('',*,*,#3250,.T.);
#4186=ORIENTED_EDGE('',*,*,#3251,.F.);
#4187=ORIENTED_EDGE('',*,*,#3213,.F.);
#4188=ORIENTED_EDGE('',*,*,#3251,.T.);
#4189=ORIENTED_EDGE('',*,*,#3252,.T.);
#4190=ORIENTED_EDGE('',*,*,#3253,.F.);
#4191=ORIENTED_EDGE('',*,*,#3254,.T.);
#4192=ORIENTED_EDGE('',*,*,#3255,.F.);
#4193=ORIENTED_EDGE('',*,*,#3214,.F.);
#4194=ORIENTED_EDGE('',*,*,#3253,.T.);
#4195=ORIENTED_EDGE('',*,*,#3246,.F.);
#4196=ORIENTED_EDGE('',*,*,#3256,.F.);
#4197=ORIENTED_EDGE('',*,*,#3257,.F.);
#4198=ORIENTED_EDGE('',*,*,#3258,.F.);
#4199=ORIENTED_EDGE('',*,*,#3250,.F.);
#4200=ORIENTED_EDGE('',*,*,#3254,.F.);
#4201=ORIENTED_EDGE('',*,*,#3259,.F.);
#4202=ORIENTED_EDGE('',*,*,#3260,.F.);
#4203=ORIENTED_EDGE('',*,*,#3261,.T.);
#4204=ORIENTED_EDGE('',*,*,#3259,.T.);
#4205=ORIENTED_EDGE('',*,*,#3252,.F.);
#4206=ORIENTED_EDGE('',*,*,#3258,.T.);
#4207=ORIENTED_EDGE('',*,*,#3262,.T.);
#4208=ORIENTED_EDGE('',*,*,#3263,.F.);
#4209=ORIENTED_EDGE('',*,*,#3264,.F.);
#4210=ORIENTED_EDGE('',*,*,#3262,.F.);
#4211=ORIENTED_EDGE('',*,*,#3257,.T.);
#4212=ORIENTED_EDGE('',*,*,#3265,.F.);
#4213=ORIENTED_EDGE('',*,*,#3237,.F.);
#4214=ORIENTED_EDGE('',*,*,#3266,.T.);
#4215=ORIENTED_EDGE('',*,*,#3265,.T.);
#4216=ORIENTED_EDGE('',*,*,#3267,.F.);
#4217=ORIENTED_EDGE('',*,*,#3256,.T.);
#4218=ORIENTED_EDGE('',*,*,#3268,.F.);
#4219=ORIENTED_EDGE('',*,*,#3238,.F.);
#4220=ORIENTED_EDGE('',*,*,#3267,.T.);
#4221=ORIENTED_EDGE('',*,*,#3268,.T.);
#4222=ORIENTED_EDGE('',*,*,#3245,.T.);
#4223=ORIENTED_EDGE('',*,*,#3241,.T.);
#4224=ORIENTED_EDGE('',*,*,#3236,.F.);
#4225=ORIENTED_EDGE('',*,*,#3269,.F.);
#4226=ORIENTED_EDGE('',*,*,#3260,.T.);
#4227=ORIENTED_EDGE('',*,*,#3266,.F.);
#4228=ORIENTED_EDGE('',*,*,#3269,.T.);
#4229=ORIENTED_EDGE('',*,*,#3270,.T.);
#4230=ORIENTED_EDGE('',*,*,#3271,.T.);
#4231=ORIENTED_EDGE('',*,*,#3261,.F.);
#4232=ORIENTED_EDGE('',*,*,#3271,.F.);
#4233=ORIENTED_EDGE('',*,*,#3272,.T.);
#4234=ORIENTED_EDGE('',*,*,#3273,.F.);
#4235=ORIENTED_EDGE('',*,*,#3274,.T.);
#4236=ORIENTED_EDGE('',*,*,#3255,.T.);
#4237=ORIENTED_EDGE('',*,*,#3273,.T.);
#4238=ORIENTED_EDGE('',*,*,#3275,.T.);
#4239=ORIENTED_EDGE('',*,*,#3276,.F.);
#4240=ORIENTED_EDGE('',*,*,#3215,.F.);
#4241=ORIENTED_EDGE('',*,*,#3274,.F.);
#4242=ORIENTED_EDGE('',*,*,#3272,.F.);
#4243=ORIENTED_EDGE('',*,*,#3277,.F.);
#4244=ORIENTED_EDGE('',*,*,#3278,.T.);
#4245=ORIENTED_EDGE('',*,*,#3275,.F.);
#4246=ORIENTED_EDGE('',*,*,#3278,.F.);
#4247=ORIENTED_EDGE('',*,*,#3279,.F.);
#4248=ORIENTED_EDGE('',*,*,#3280,.T.);
#4249=ORIENTED_EDGE('',*,*,#3281,.F.);
#4250=ORIENTED_EDGE('',*,*,#3281,.T.);
#4251=ORIENTED_EDGE('',*,*,#3282,.T.);
#4252=ORIENTED_EDGE('',*,*,#3276,.T.);
#4253=ORIENTED_EDGE('',*,*,#3210,.F.);
#4254=ORIENTED_EDGE('',*,*,#3282,.F.);
#4255=ORIENTED_EDGE('',*,*,#3283,.T.);
#4256=ORIENTED_EDGE('',*,*,#3284,.F.);
#4257=ORIENTED_EDGE('',*,*,#3285,.T.);
#4258=ORIENTED_EDGE('',*,*,#3284,.T.);
#4259=ORIENTED_EDGE('',*,*,#3286,.T.);
#4260=ORIENTED_EDGE('',*,*,#3211,.F.);
#4261=ORIENTED_EDGE('',*,*,#3285,.F.);
#4262=ORIENTED_EDGE('',*,*,#3243,.T.);
#4263=ORIENTED_EDGE('',*,*,#3249,.F.);
#4264=ORIENTED_EDGE('',*,*,#3287,.F.);
#4265=ORIENTED_EDGE('',*,*,#3288,.F.);
#4266=ORIENTED_EDGE('',*,*,#3244,.T.);
#4267=ORIENTED_EDGE('',*,*,#3286,.F.);
#4268=ORIENTED_EDGE('',*,*,#3289,.F.);
#4269=ORIENTED_EDGE('',*,*,#3287,.T.);
#4270=ORIENTED_EDGE('',*,*,#3283,.F.);
#4271=ORIENTED_EDGE('',*,*,#3280,.F.);
#4272=ORIENTED_EDGE('',*,*,#3290,.F.);
#4273=ORIENTED_EDGE('',*,*,#3289,.T.);
#4274=ORIENTED_EDGE('',*,*,#3291,.F.);
#4275=ORIENTED_EDGE('',*,*,#3234,.F.);
#4276=ORIENTED_EDGE('',*,*,#3292,.F.);
#4277=ORIENTED_EDGE('',*,*,#3288,.T.);
#4278=ORIENTED_EDGE('',*,*,#3292,.T.);
#4279=ORIENTED_EDGE('',*,*,#3240,.T.);
#4280=ORIENTED_EDGE('',*,*,#3293,.T.);
#4281=ORIENTED_EDGE('',*,*,#3291,.T.);
#4282=ORIENTED_EDGE('',*,*,#3279,.T.);
#4283=ORIENTED_EDGE('',*,*,#3235,.F.);
#4284=ORIENTED_EDGE('',*,*,#3293,.F.);
#4285=ORIENTED_EDGE('',*,*,#3277,.T.);
#4286=ORIENTED_EDGE('',*,*,#3270,.F.);
#4287=ORIENTED_EDGE('',*,*,#3294,.F.);
#4288=ORIENTED_EDGE('',*,*,#3295,.T.);
#4289=ORIENTED_EDGE('',*,*,#3290,.T.);
#4290=ORIENTED_EDGE('',*,*,#3295,.F.);
#4291=ORIENTED_EDGE('',*,*,#3294,.T.);
#4292=ORIENTED_EDGE('',*,*,#3296,.F.);
#4293=ORIENTED_EDGE('',*,*,#3297,.F.);
#4294=ORIENTED_EDGE('',*,*,#3298,.T.);
#4295=ORIENTED_EDGE('',*,*,#3296,.T.);
#4296=ORIENTED_EDGE('',*,*,#3298,.F.);
#4297=ORIENTED_EDGE('',*,*,#3225,.F.);
#4298=ORIENTED_EDGE('',*,*,#3226,.F.);
#4299=ORIENTED_EDGE('',*,*,#3299,.T.);
#4300=ORIENTED_EDGE('',*,*,#3297,.T.);
#4301=ORIENTED_EDGE('',*,*,#3299,.F.);
#4302=ORIENTED_EDGE('',*,*,#3300,.T.);
#4303=ORIENTED_EDGE('',*,*,#3301,.T.);
#4304=ORIENTED_EDGE('',*,*,#3263,.T.);
#4305=ORIENTED_EDGE('',*,*,#3264,.T.);
#4306=ORIENTED_EDGE('',*,*,#3301,.F.);
#4307=ORIENTED_EDGE('',*,*,#3302,.T.);
#4308=ORIENTED_EDGE('',*,*,#3303,.T.);
#4309=ORIENTED_EDGE('',*,*,#3304,.T.);
#4310=ORIENTED_EDGE('',*,*,#3305,.T.);
#4311=ORIENTED_EDGE('',*,*,#3306,.F.);
#4312=ORIENTED_EDGE('',*,*,#3307,.F.);
#4313=ORIENTED_EDGE('',*,*,#3305,.F.);
#4314=ORIENTED_EDGE('',*,*,#3300,.F.);
#4315=ORIENTED_EDGE('',*,*,#3308,.T.);
#4316=ORIENTED_EDGE('',*,*,#3306,.T.);
#4317=ORIENTED_EDGE('',*,*,#3307,.T.);
#4318=ORIENTED_EDGE('',*,*,#3308,.F.);
#4319=ORIENTED_EDGE('',*,*,#3302,.F.);
#4320=ORIENTED_EDGE('',*,*,#3303,.F.);
#4321=ORIENTED_EDGE('',*,*,#3304,.F.);
#4322=ORIENTED_EDGE('',*,*,#3309,.T.);
#4323=ORIENTED_EDGE('',*,*,#3310,.F.);
#4324=ORIENTED_EDGE('',*,*,#3311,.T.);
#4325=ORIENTED_EDGE('',*,*,#3312,.T.);
#4326=ORIENTED_EDGE('',*,*,#3313,.T.);
#4327=ORIENTED_EDGE('',*,*,#3314,.T.);
#4328=ORIENTED_EDGE('',*,*,#3315,.T.);
#4329=ORIENTED_EDGE('',*,*,#3316,.T.);
#4330=ORIENTED_EDGE('',*,*,#3317,.F.);
#4331=ORIENTED_EDGE('',*,*,#3318,.T.);
#4332=ORIENTED_EDGE('',*,*,#3319,.F.);
#4333=ORIENTED_EDGE('',*,*,#3309,.F.);
#4334=ORIENTED_EDGE('',*,*,#3320,.F.);
#4335=ORIENTED_EDGE('',*,*,#3321,.T.);
#4336=ORIENTED_EDGE('',*,*,#3317,.T.);
#4337=ORIENTED_EDGE('',*,*,#3322,.F.);
#4338=ORIENTED_EDGE('',*,*,#3323,.T.);
#4339=ORIENTED_EDGE('',*,*,#3320,.T.);
#4340=ORIENTED_EDGE('',*,*,#3324,.T.);
#4341=ORIENTED_EDGE('',*,*,#3325,.F.);
#4342=ORIENTED_EDGE('',*,*,#3326,.T.);
#4343=ORIENTED_EDGE('',*,*,#3327,.T.);
#4344=ORIENTED_EDGE('',*,*,#3328,.F.);
#4345=ORIENTED_EDGE('',*,*,#3329,.T.);
#4346=ORIENTED_EDGE('',*,*,#3330,.T.);
#4347=ORIENTED_EDGE('',*,*,#3331,.F.);
#4348=ORIENTED_EDGE('',*,*,#3332,.F.);
#4349=ORIENTED_EDGE('',*,*,#3333,.T.);
#4350=ORIENTED_EDGE('',*,*,#3333,.F.);
#4351=ORIENTED_EDGE('',*,*,#3334,.T.);
#4352=ORIENTED_EDGE('',*,*,#3335,.F.);
#4353=ORIENTED_EDGE('',*,*,#3336,.F.);
#4354=ORIENTED_EDGE('',*,*,#3337,.T.);
#4355=ORIENTED_EDGE('',*,*,#3338,.T.);
#4356=ORIENTED_EDGE('',*,*,#3337,.F.);
#4357=ORIENTED_EDGE('',*,*,#3339,.F.);
#4358=ORIENTED_EDGE('',*,*,#3334,.F.);
#4359=ORIENTED_EDGE('',*,*,#3338,.F.);
#4360=ORIENTED_EDGE('',*,*,#3336,.T.);
#4361=ORIENTED_EDGE('',*,*,#3340,.T.);
#4362=ORIENTED_EDGE('',*,*,#3341,.T.);
#4363=ORIENTED_EDGE('',*,*,#3340,.F.);
#4364=ORIENTED_EDGE('',*,*,#3335,.T.);
#4365=ORIENTED_EDGE('',*,*,#3339,.T.);
#4366=ORIENTED_EDGE('',*,*,#3342,.T.);
#4367=ORIENTED_EDGE('',*,*,#3332,.T.);
#4368=ORIENTED_EDGE('',*,*,#3343,.T.);
#4369=ORIENTED_EDGE('',*,*,#3344,.T.);
#4370=ORIENTED_EDGE('',*,*,#3345,.T.);
#4371=ORIENTED_EDGE('',*,*,#3346,.T.);
#4372=ORIENTED_EDGE('',*,*,#3310,.T.);
#4373=ORIENTED_EDGE('',*,*,#3319,.T.);
#4374=ORIENTED_EDGE('',*,*,#3347,.T.);
#4375=ORIENTED_EDGE('',*,*,#3348,.T.);
#4376=ORIENTED_EDGE('',*,*,#3349,.T.);
#4377=ORIENTED_EDGE('',*,*,#3350,.F.);
#4378=ORIENTED_EDGE('',*,*,#3328,.T.);
#4379=ORIENTED_EDGE('',*,*,#3351,.F.);
#4380=ORIENTED_EDGE('',*,*,#3352,.T.);
#4381=ORIENTED_EDGE('',*,*,#3353,.T.);
#4382=ORIENTED_EDGE('',*,*,#3354,.T.);
#4383=ORIENTED_EDGE('',*,*,#3355,.T.);
#4384=ORIENTED_EDGE('',*,*,#3356,.T.);
#4385=ORIENTED_EDGE('',*,*,#3357,.F.);
#4386=ORIENTED_EDGE('',*,*,#3358,.F.);
#4387=ORIENTED_EDGE('',*,*,#3341,.F.);
#4388=ORIENTED_EDGE('',*,*,#3359,.T.);
#4389=ORIENTED_EDGE('',*,*,#3360,.T.);
#4390=ORIENTED_EDGE('',*,*,#3358,.T.);
#4391=ORIENTED_EDGE('',*,*,#3360,.F.);
#4392=ORIENTED_EDGE('',*,*,#3361,.T.);
#4393=ORIENTED_EDGE('',*,*,#3362,.T.);
#4394=ORIENTED_EDGE('',*,*,#3363,.T.);
#4395=ORIENTED_EDGE('',*,*,#3364,.F.);
#4396=ORIENTED_EDGE('',*,*,#3365,.T.);
#4397=ORIENTED_EDGE('',*,*,#3361,.F.);
#4398=ORIENTED_EDGE('',*,*,#3359,.F.);
#4399=ORIENTED_EDGE('',*,*,#3363,.F.);
#4400=ORIENTED_EDGE('',*,*,#3366,.T.);
#4401=ORIENTED_EDGE('',*,*,#3367,.T.);
#4402=ORIENTED_EDGE('',*,*,#3366,.F.);
#4403=ORIENTED_EDGE('',*,*,#3362,.F.);
#4404=ORIENTED_EDGE('',*,*,#3365,.F.);
#4405=ORIENTED_EDGE('',*,*,#3368,.F.);
#4406=ORIENTED_EDGE('',*,*,#3369,.F.);
#4407=ORIENTED_EDGE('',*,*,#3370,.F.);
#4408=ORIENTED_EDGE('',*,*,#3371,.F.);
#4409=ORIENTED_EDGE('',*,*,#3372,.F.);
#4410=ORIENTED_EDGE('',*,*,#3373,.F.);
#4411=ORIENTED_EDGE('',*,*,#3344,.F.);
#4412=ORIENTED_EDGE('',*,*,#3374,.T.);
#4413=ORIENTED_EDGE('',*,*,#3375,.F.);
#4414=ORIENTED_EDGE('',*,*,#3376,.F.);
#4415=ORIENTED_EDGE('',*,*,#3349,.F.);
#4416=ORIENTED_EDGE('',*,*,#3377,.T.);
#4417=ORIENTED_EDGE('',*,*,#3367,.F.);
#4418=ORIENTED_EDGE('',*,*,#3364,.T.);
#4419=ORIENTED_EDGE('',*,*,#3368,.T.);
#4420=ORIENTED_EDGE('',*,*,#3378,.F.);
#4421=ORIENTED_EDGE('',*,*,#3379,.F.);
#4422=ORIENTED_EDGE('',*,*,#3380,.F.);
#4423=ORIENTED_EDGE('',*,*,#3381,.F.);
#4424=ORIENTED_EDGE('',*,*,#3382,.F.);
#4425=ORIENTED_EDGE('',*,*,#3383,.T.);
#4426=ORIENTED_EDGE('',*,*,#3381,.T.);
#4427=ORIENTED_EDGE('',*,*,#3384,.T.);
#4428=ORIENTED_EDGE('',*,*,#3385,.T.);
#4429=ORIENTED_EDGE('',*,*,#3386,.F.);
#4430=ORIENTED_EDGE('',*,*,#3315,.F.);
#4431=ORIENTED_EDGE('',*,*,#3387,.F.);
#4432=ORIENTED_EDGE('',*,*,#3388,.T.);
#4433=ORIENTED_EDGE('',*,*,#3382,.T.);
#4434=ORIENTED_EDGE('',*,*,#3389,.T.);
#4435=ORIENTED_EDGE('',*,*,#3390,.T.);
#4436=ORIENTED_EDGE('',*,*,#3391,.F.);
#4437=ORIENTED_EDGE('',*,*,#3392,.T.);
#4438=ORIENTED_EDGE('',*,*,#3393,.T.);
#4439=ORIENTED_EDGE('',*,*,#3394,.T.);
#4440=ORIENTED_EDGE('',*,*,#3395,.F.);
#4441=ORIENTED_EDGE('',*,*,#3395,.T.);
#4442=ORIENTED_EDGE('',*,*,#3396,.T.);
#4443=ORIENTED_EDGE('',*,*,#3348,.F.);
#4444=ORIENTED_EDGE('',*,*,#3396,.F.);
#4445=ORIENTED_EDGE('',*,*,#3385,.F.);
#4446=ORIENTED_EDGE('',*,*,#3397,.F.);
#4447=ORIENTED_EDGE('',*,*,#3325,.T.);
#4448=ORIENTED_EDGE('',*,*,#3398,.T.);
#4449=ORIENTED_EDGE('',*,*,#3399,.T.);
#4450=ORIENTED_EDGE('',*,*,#3398,.F.);
#4451=ORIENTED_EDGE('',*,*,#3324,.F.);
#4452=ORIENTED_EDGE('',*,*,#3322,.T.);
#4453=ORIENTED_EDGE('',*,*,#3400,.F.);
#4454=ORIENTED_EDGE('',*,*,#3347,.F.);
#4455=ORIENTED_EDGE('',*,*,#3318,.F.);
#4456=ORIENTED_EDGE('',*,*,#3399,.F.);
#4457=ORIENTED_EDGE('',*,*,#3316,.F.);
#4458=ORIENTED_EDGE('',*,*,#3386,.T.);
#4459=ORIENTED_EDGE('',*,*,#3401,.T.);
#4460=ORIENTED_EDGE('',*,*,#3311,.F.);
#4461=ORIENTED_EDGE('',*,*,#3346,.F.);
#4462=ORIENTED_EDGE('',*,*,#3402,.T.);
#4463=ORIENTED_EDGE('',*,*,#3387,.T.);
#4464=ORIENTED_EDGE('',*,*,#3314,.F.);
#4465=ORIENTED_EDGE('',*,*,#3342,.F.);
#4466=ORIENTED_EDGE('',*,*,#3400,.T.);
#4467=ORIENTED_EDGE('',*,*,#3321,.F.);
#4468=ORIENTED_EDGE('',*,*,#3323,.F.);
#4469=ORIENTED_EDGE('',*,*,#3345,.F.);
#4470=ORIENTED_EDGE('',*,*,#3373,.T.);
#4471=ORIENTED_EDGE('',*,*,#3403,.F.);
#4472=ORIENTED_EDGE('',*,*,#3401,.F.);
#4473=ORIENTED_EDGE('',*,*,#3312,.F.);
#4474=ORIENTED_EDGE('',*,*,#3403,.T.);
#4475=ORIENTED_EDGE('',*,*,#3372,.T.);
#4476=ORIENTED_EDGE('',*,*,#3404,.F.);
#4477=ORIENTED_EDGE('',*,*,#3313,.F.);
#4478=ORIENTED_EDGE('',*,*,#3404,.T.);
#4479=ORIENTED_EDGE('',*,*,#3371,.T.);
#4480=ORIENTED_EDGE('',*,*,#3405,.F.);
#4481=ORIENTED_EDGE('',*,*,#3370,.T.);
#4482=ORIENTED_EDGE('',*,*,#3406,.T.);
#4483=ORIENTED_EDGE('',*,*,#3402,.F.);
#4484=ORIENTED_EDGE('',*,*,#3405,.T.);
#4485=ORIENTED_EDGE('',*,*,#3388,.F.);
#4486=ORIENTED_EDGE('',*,*,#3406,.F.);
#4487=ORIENTED_EDGE('',*,*,#3369,.T.);
#4488=ORIENTED_EDGE('',*,*,#3383,.F.);
#4489=ORIENTED_EDGE('',*,*,#3394,.F.);
#4490=ORIENTED_EDGE('',*,*,#3407,.T.);
#4491=ORIENTED_EDGE('',*,*,#3408,.T.);
#4492=ORIENTED_EDGE('',*,*,#3397,.T.);
#4493=ORIENTED_EDGE('',*,*,#3409,.T.);
#4494=ORIENTED_EDGE('',*,*,#3410,.T.);
#4495=ORIENTED_EDGE('',*,*,#3411,.F.);
#4496=ORIENTED_EDGE('',*,*,#3326,.F.);
#4497=ORIENTED_EDGE('',*,*,#3408,.F.);
#4498=ORIENTED_EDGE('',*,*,#3412,.F.);
#4499=ORIENTED_EDGE('',*,*,#3409,.F.);
#4500=ORIENTED_EDGE('',*,*,#3413,.F.);
#4501=ORIENTED_EDGE('',*,*,#3414,.F.);
#4502=ORIENTED_EDGE('',*,*,#3415,.F.);
#4503=ORIENTED_EDGE('',*,*,#3410,.F.);
#4504=ORIENTED_EDGE('',*,*,#3416,.F.);
#4505=ORIENTED_EDGE('',*,*,#3417,.F.);
#4506=ORIENTED_EDGE('',*,*,#3418,.T.);
#4507=ORIENTED_EDGE('',*,*,#3416,.T.);
#4508=ORIENTED_EDGE('',*,*,#3412,.T.);
#4509=ORIENTED_EDGE('',*,*,#3418,.F.);
#4510=ORIENTED_EDGE('',*,*,#3419,.T.);
#4511=ORIENTED_EDGE('',*,*,#3420,.F.);
#4512=ORIENTED_EDGE('',*,*,#3421,.T.);
#4513=ORIENTED_EDGE('',*,*,#3391,.T.);
#4514=ORIENTED_EDGE('',*,*,#3422,.T.);
#4515=ORIENTED_EDGE('',*,*,#3423,.T.);
#4516=ORIENTED_EDGE('',*,*,#3424,.T.);
#4517=ORIENTED_EDGE('',*,*,#3354,.F.);
#4518=ORIENTED_EDGE('',*,*,#3417,.T.);
#4519=ORIENTED_EDGE('',*,*,#3425,.T.);
#4520=ORIENTED_EDGE('',*,*,#3425,.F.);
#4521=ORIENTED_EDGE('',*,*,#3426,.T.);
#4522=ORIENTED_EDGE('',*,*,#3427,.T.);
#4523=ORIENTED_EDGE('',*,*,#3426,.F.);
#4524=ORIENTED_EDGE('',*,*,#3427,.F.);
#4525=ORIENTED_EDGE('',*,*,#3379,.T.);
#4526=ORIENTED_EDGE('',*,*,#3428,.F.);
#4527=ORIENTED_EDGE('',*,*,#3429,.T.);
#4528=ORIENTED_EDGE('',*,*,#3430,.F.);
#4529=ORIENTED_EDGE('',*,*,#3380,.T.);
#4530=ORIENTED_EDGE('',*,*,#3389,.F.);
#4531=ORIENTED_EDGE('',*,*,#3384,.F.);
#4532=ORIENTED_EDGE('',*,*,#3430,.T.);
#4533=ORIENTED_EDGE('',*,*,#3431,.F.);
#4534=ORIENTED_EDGE('',*,*,#3432,.T.);
#4535=ORIENTED_EDGE('',*,*,#3431,.T.);
#4536=ORIENTED_EDGE('',*,*,#3433,.T.);
#4537=ORIENTED_EDGE('',*,*,#3422,.F.);
#4538=ORIENTED_EDGE('',*,*,#3390,.F.);
#4539=ORIENTED_EDGE('',*,*,#3432,.F.);
#4540=ORIENTED_EDGE('',*,*,#3434,.T.);
#4541=ORIENTED_EDGE('',*,*,#3435,.F.);
#4542=ORIENTED_EDGE('',*,*,#3423,.F.);
#4543=ORIENTED_EDGE('',*,*,#3434,.F.);
#4544=ORIENTED_EDGE('',*,*,#3436,.F.);
#4545=ORIENTED_EDGE('',*,*,#3424,.F.);
#4546=ORIENTED_EDGE('',*,*,#3435,.T.);
#4547=ORIENTED_EDGE('',*,*,#3437,.F.);
#4548=ORIENTED_EDGE('',*,*,#3355,.F.);
#4549=ORIENTED_EDGE('',*,*,#3438,.T.);
#4550=ORIENTED_EDGE('',*,*,#3437,.T.);
#4551=ORIENTED_EDGE('',*,*,#3439,.T.);
#4552=ORIENTED_EDGE('',*,*,#3428,.T.);
#4553=ORIENTED_EDGE('',*,*,#3440,.F.);
#4554=ORIENTED_EDGE('',*,*,#3356,.F.);
#4555=ORIENTED_EDGE('',*,*,#3438,.F.);
#4556=ORIENTED_EDGE('',*,*,#3377,.F.);
#4557=ORIENTED_EDGE('',*,*,#3357,.T.);
#4558=ORIENTED_EDGE('',*,*,#3440,.T.);
#4559=ORIENTED_EDGE('',*,*,#3378,.T.);
#4560=ORIENTED_EDGE('',*,*,#3429,.F.);
#4561=ORIENTED_EDGE('',*,*,#3439,.F.);
#4562=ORIENTED_EDGE('',*,*,#3436,.T.);
#4563=ORIENTED_EDGE('',*,*,#3433,.F.);
#4564=ORIENTED_EDGE('',*,*,#3419,.F.);
#4565=ORIENTED_EDGE('',*,*,#3353,.F.);
#4566=ORIENTED_EDGE('',*,*,#3441,.F.);
#4567=ORIENTED_EDGE('',*,*,#3442,.T.);
#4568=ORIENTED_EDGE('',*,*,#3442,.F.);
#4569=ORIENTED_EDGE('',*,*,#3443,.T.);
#4570=ORIENTED_EDGE('',*,*,#3444,.F.);
#4571=ORIENTED_EDGE('',*,*,#3420,.T.);
#4572=ORIENTED_EDGE('',*,*,#3421,.F.);
#4573=ORIENTED_EDGE('',*,*,#3444,.T.);
#4574=ORIENTED_EDGE('',*,*,#3445,.F.);
#4575=ORIENTED_EDGE('',*,*,#3392,.F.);
#4576=ORIENTED_EDGE('',*,*,#3445,.T.);
#4577=ORIENTED_EDGE('',*,*,#3446,.T.);
#4578=ORIENTED_EDGE('',*,*,#3447,.T.);
#4579=ORIENTED_EDGE('',*,*,#3393,.F.);
#4580=ORIENTED_EDGE('',*,*,#3447,.F.);
#4581=ORIENTED_EDGE('',*,*,#3413,.T.);
#4582=ORIENTED_EDGE('',*,*,#3407,.F.);
#4583=ORIENTED_EDGE('',*,*,#3443,.F.);
#4584=ORIENTED_EDGE('',*,*,#3448,.F.);
#4585=ORIENTED_EDGE('',*,*,#3414,.T.);
#4586=ORIENTED_EDGE('',*,*,#3446,.F.);
#4587=ORIENTED_EDGE('',*,*,#3448,.T.);
#4588=ORIENTED_EDGE('',*,*,#3441,.T.);
#4589=ORIENTED_EDGE('',*,*,#3449,.T.);
#4590=ORIENTED_EDGE('',*,*,#3415,.T.);
#4591=ORIENTED_EDGE('',*,*,#3449,.F.);
#4592=ORIENTED_EDGE('',*,*,#3352,.F.);
#4593=ORIENTED_EDGE('',*,*,#3450,.F.);
#4594=ORIENTED_EDGE('',*,*,#3327,.F.);
#4595=ORIENTED_EDGE('',*,*,#3411,.T.);
#4596=ORIENTED_EDGE('',*,*,#3450,.T.);
#4597=ORIENTED_EDGE('',*,*,#3351,.T.);
#4598=ORIENTED_EDGE('',*,*,#3350,.T.);
#4599=ORIENTED_EDGE('',*,*,#3376,.T.);
#4600=ORIENTED_EDGE('',*,*,#3451,.F.);
#4601=ORIENTED_EDGE('',*,*,#3329,.F.);
#4602=ORIENTED_EDGE('',*,*,#3375,.T.);
#4603=ORIENTED_EDGE('',*,*,#3452,.F.);
#4604=ORIENTED_EDGE('',*,*,#3330,.F.);
#4605=ORIENTED_EDGE('',*,*,#3451,.T.);
#4606=ORIENTED_EDGE('',*,*,#3343,.F.);
#4607=ORIENTED_EDGE('',*,*,#3331,.T.);
#4608=ORIENTED_EDGE('',*,*,#3452,.T.);
#4609=ORIENTED_EDGE('',*,*,#3374,.F.);
#4610=ORIENTED_EDGE('',*,*,#3453,.F.);
#4611=ORIENTED_EDGE('',*,*,#3454,.T.);
#4612=ORIENTED_EDGE('',*,*,#3455,.T.);
#4613=ORIENTED_EDGE('',*,*,#3454,.F.);
#4614=ORIENTED_EDGE('',*,*,#3455,.F.);
#4615=ORIENTED_EDGE('',*,*,#3456,.F.);
#4616=ORIENTED_EDGE('',*,*,#3457,.F.);
#4617=ORIENTED_EDGE('',*,*,#3458,.T.);
#4618=ORIENTED_EDGE('',*,*,#3459,.T.);
#4619=ORIENTED_EDGE('',*,*,#3458,.F.);
#4620=ORIENTED_EDGE('',*,*,#3459,.F.);
#4621=ORIENTED_EDGE('',*,*,#3460,.F.);
#5528=PLANE('',#6302);
#5529=PLANE('',#6310);
#5530=PLANE('',#6314);
#5531=PLANE('',#6322);
#5532=PLANE('',#6326);
#5533=PLANE('',#6338);
#5534=PLANE('',#6341);
#5535=PLANE('',#6363);
#5536=PLANE('',#6377);
#5537=PLANE('',#6388);
#5538=PLANE('',#6411);
#5539=PLANE('',#6416);
#5540=PLANE('',#6419);
#5541=PLANE('',#6423);
#5542=PLANE('',#6429);
#5543=PLANE('',#6431);
#5544=PLANE('',#6439);
#5545=PLANE('',#6447);
#5546=PLANE('',#6448);
#5547=PLANE('',#6449);
#5548=PLANE('',#6450);
#5549=PLANE('',#6464);
#5550=PLANE('',#6469);
#5551=PLANE('',#6477);
#5552=PLANE('',#6484);
#5553=PLANE('',#6496);
#5554=PLANE('',#6510);
#5555=PLANE('',#6511);
#5556=PLANE('',#6512);
#5557=PLANE('',#6516);
#5558=PLANE('',#6521);
#5702=ADVANCED_FACE('',(#1054,#528),#5528,.F.);
#5703=ADVANCED_FACE('',(#1055),#364,.T.);
#5704=ADVANCED_FACE('',(#1056),#126,.T.);
#5705=ADVANCED_FACE('',(#1057,#529),#5529,.F.);
#5706=ADVANCED_FACE('',(#1058,#530),#365,.F.);
#5707=ADVANCED_FACE('',(#1059,#531),#5530,.T.);
#5708=ADVANCED_FACE('',(#1060),#127,.T.);
#5709=ADVANCED_FACE('',(#1061),#366,.T.);
#5710=ADVANCED_FACE('',(#1062,#532),#5531,.T.);
#5711=ADVANCED_FACE('',(#1063),#367,.T.);
#5712=ADVANCED_FACE('',(#1064),#5532,.T.);
#5713=ADVANCED_FACE('',(#1065),#368,.T.);
#5714=ADVANCED_FACE('',(#1066),#114,.T.);
#5715=ADVANCED_FACE('',(#1067),#369,.T.);
#5716=ADVANCED_FACE('',(#1068),#109,.T.);
#5717=ADVANCED_FACE('',(#1069),#370,.T.);
#5718=ADVANCED_FACE('',(#1070),#5533,.T.);
#5719=ADVANCED_FACE('',(#1071),#5534,.T.);
#5720=ADVANCED_FACE('',(#1072),#128,.F.);
#5721=ADVANCED_FACE('',(#1073),#110,.T.);
#5722=ADVANCED_FACE('',(#1074),#371,.T.);
#5723=ADVANCED_FACE('',(#1075),#115,.T.);
#5724=ADVANCED_FACE('',(#1076),#372,.T.);
#5725=ADVANCED_FACE('',(#1077),#116,.T.);
#5726=ADVANCED_FACE('',(#1078),#373,.T.);
#5727=ADVANCED_FACE('',(#1079),#117,.T.);
#5728=ADVANCED_FACE('',(#1080),#374,.T.);
#5729=ADVANCED_FACE('',(#1081),#5535,.T.);
#5730=ADVANCED_FACE('',(#1082),#375,.T.);
#5731=ADVANCED_FACE('',(#1083),#118,.T.);
#5732=ADVANCED_FACE('',(#1084),#376,.T.);
#5733=ADVANCED_FACE('',(#1085),#119,.T.);
#5734=ADVANCED_FACE('',(#1086),#377,.T.);
#5735=ADVANCED_FACE('',(#1087),#378,.T.);
#5736=ADVANCED_FACE('',(#1088,#533),#5536,.T.);
#5737=ADVANCED_FACE('',(#1089),#379,.T.);
#5738=ADVANCED_FACE('',(#1090),#120,.T.);
#5739=ADVANCED_FACE('',(#1091),#121,.T.);
#5740=ADVANCED_FACE('',(#1092),#380,.T.);
#5741=ADVANCED_FACE('',(#1093),#381,.T.);
#5742=ADVANCED_FACE('',(#1094,#534),#5537,.T.);
#5743=ADVANCED_FACE('',(#1095),#261,.F.);
#5744=ADVANCED_FACE('',(#1096),#382,.F.);
#5745=ADVANCED_FACE('',(#1097),#262,.T.);
#5746=ADVANCED_FACE('',(#1098),#263,.T.);
#5747=ADVANCED_FACE('',(#1099),#129,.T.);
#5748=ADVANCED_FACE('',(#1100),#130,.F.);
#5749=ADVANCED_FACE('',(#1101),#111,.T.);
#5750=ADVANCED_FACE('',(#1102,#535),#5538,.T.);
#5751=ADVANCED_FACE('',(#1103),#383,.F.);
#5752=ADVANCED_FACE('',(#1104),#5539,.F.);
#5753=ADVANCED_FACE('',(#1105),#384,.F.);
#5754=ADVANCED_FACE('',(#1106,#536),#5540,.T.);
#5755=ADVANCED_FACE('',(#1107,#537,#538),#5541,.T.);
#5756=ADVANCED_FACE('',(#1108),#385,.F.);
#5757=ADVANCED_FACE('',(#1109),#386,.F.);
#5758=ADVANCED_FACE('',(#1110,#539),#5542,.T.);
#5759=ADVANCED_FACE('',(#1111),#5543,.T.);
#5760=ADVANCED_FACE('',(#1112),#387,.F.);
#5761=ADVANCED_FACE('',(#1113),#131,.T.);
#5762=ADVANCED_FACE('',(#1114,#540),#5544,.F.);
#5763=ADVANCED_FACE('',(#1115),#388,.F.);
#5764=ADVANCED_FACE('',(#1116),#389,.T.);
#5765=ADVANCED_FACE('',(#1117),#390,.T.);
#5766=ADVANCED_FACE('',(#1118),#5545,.T.);
#5767=ADVANCED_FACE('',(#1119),#5546,.T.);
#5768=ADVANCED_FACE('',(#1120),#5547,.T.);
#5769=ADVANCED_FACE('',(#1121),#5548,.T.);
#5770=ADVANCED_FACE('',(#1122),#391,.T.);
#5771=ADVANCED_FACE('',(#1123),#392,.T.);
#5772=ADVANCED_FACE('',(#1124),#112,.T.);
#5773=ADVANCED_FACE('',(#1125),#113,.T.);
#5774=ADVANCED_FACE('',(#1126),#393,.T.);
#5775=ADVANCED_FACE('',(#1127),#394,.T.);
#5776=ADVANCED_FACE('',(#1128),#132,.T.);
#5777=ADVANCED_FACE('',(#1129),#395,.F.);
#5778=ADVANCED_FACE('',(#1130),#5549,.T.);
#5779=ADVANCED_FACE('',(#1131),#396,.F.);
#5780=ADVANCED_FACE('',(#1132,#541,#542),#5550,.T.);
#5781=ADVANCED_FACE('',(#1133),#397,.F.);
#5782=ADVANCED_FACE('',(#1134),#5551,.T.);
#5783=ADVANCED_FACE('',(#1135),#398,.T.);
#5784=ADVANCED_FACE('',(#1136),#122,.T.);
#5785=ADVANCED_FACE('',(#1137),#399,.T.);
#5786=ADVANCED_FACE('',(#1138),#5552,.T.);
#5787=ADVANCED_FACE('',(#1139),#400,.T.);
#5788=ADVANCED_FACE('',(#1140),#123,.T.);
#5789=ADVANCED_FACE('',(#1141),#401,.T.);
#5790=ADVANCED_FACE('',(#1142),#133,.F.);
#5791=ADVANCED_FACE('',(#1143),#402,.T.);
#5792=ADVANCED_FACE('',(#1144),#403,.T.);
#5793=ADVANCED_FACE('',(#1145),#5553,.T.);
#5794=ADVANCED_FACE('',(#1146),#404,.T.);
#5795=ADVANCED_FACE('',(#1147),#124,.T.);
#5796=ADVANCED_FACE('',(#1148),#405,.T.);
#5797=ADVANCED_FACE('',(#1149),#406,.T.);
#5798=ADVANCED_FACE('',(#1150),#125,.T.);
#5799=ADVANCED_FACE('',(#1151),#407,.T.);
#5800=ADVANCED_FACE('',(#1152),#134,.F.);
#5801=ADVANCED_FACE('',(#1153),#5554,.F.);
#5802=ADVANCED_FACE('',(#1154),#5555,.F.);
#5803=ADVANCED_FACE('',(#1155),#5556,.F.);
#5804=ADVANCED_FACE('',(#1156),#408,.T.);
#5805=ADVANCED_FACE('',(#1157,#543),#5557,.F.);
#5806=ADVANCED_FACE('',(#1158),#409,.T.);
#5807=ADVANCED_FACE('',(#1159,#544),#5558,.F.);
#6018=CLOSED_SHELL('',(#5702,#5703,#5704,#5705,#5706,#5707,#5708,#5709,
#5710,#5711,#5712,#5713,#5714,#5715,#5716,#5717,#5718,#5719,#5720,#5721,
#5722,#5723,#5724,#5725,#5726,#5727,#5728,#5729,#5730,#5731,#5732,#5733,
#5734,#5735,#5736,#5737,#5738,#5739,#5740,#5741,#5742,#5743,#5744,#5745,
#5746,#5747,#5748,#5749,#5750,#5751,#5752,#5753,#5754,#5755,#5756,#5757,
#5758,#5759,#5760,#5761,#5762,#5763,#5764,#5765,#5766,#5767,#5768,#5769,
#5770,#5771,#5772,#5773,#5774,#5775,#5776,#5777,#5778,#5779,#5780,#5781,
#5782,#5783,#5784,#5785,#5786,#5787,#5788,#5789,#5790,#5791,#5792,#5793,
#5794,#5795,#5796,#5797,#5798,#5799,#5800,#5801,#5802,#5803));
#6301=AXIS2_PLACEMENT_3D('',#9101,#7226,#7227);
#6302=AXIS2_PLACEMENT_3D('',#9102,#7228,#7229);
#6303=AXIS2_PLACEMENT_3D('',#9126,#7235,#7236);
#6304=AXIS2_PLACEMENT_3D('',#9127,#7237,#7238);
#6305=AXIS2_PLACEMENT_3D('',#9131,#7240,#7241);
#6306=AXIS2_PLACEMENT_3D('',#9132,#7242,#7243);
#6307=AXIS2_PLACEMENT_3D('',#9133,#7244,#7245);
#6308=AXIS2_PLACEMENT_3D('',#9135,#7246,#7247);
#6309=AXIS2_PLACEMENT_3D('',#9136,#7248,#7249);
#6310=AXIS2_PLACEMENT_3D('',#9137,#7250,#7251);
#6311=AXIS2_PLACEMENT_3D('',#9139,#7252,#7253);
#6312=AXIS2_PLACEMENT_3D('',#9140,#7254,#7255);
#6313=AXIS2_PLACEMENT_3D('',#9143,#7257,#7258);
#6314=AXIS2_PLACEMENT_3D('',#9182,#7259,#7260);
#6315=AXIS2_PLACEMENT_3D('',#9184,#7261,#7262);
#6316=AXIS2_PLACEMENT_3D('',#9185,#7263,#7264);
#6317=AXIS2_PLACEMENT_3D('',#9187,#7265,#7266);
#6318=AXIS2_PLACEMENT_3D('',#9189,#7267,#7268);
#6319=AXIS2_PLACEMENT_3D('',#9190,#7269,#7270);
#6320=AXIS2_PLACEMENT_3D('',#9191,#7271,#7272);
#6321=AXIS2_PLACEMENT_3D('',#9194,#7274,#7275);
#6322=AXIS2_PLACEMENT_3D('',#9195,#7276,#7277);
#6323=AXIS2_PLACEMENT_3D('',#9218,#7283,#7284);
#6324=AXIS2_PLACEMENT_3D('',#9222,#7286,#7287);
#6325=AXIS2_PLACEMENT_3D('',#9223,#7288,#7289);
#6326=AXIS2_PLACEMENT_3D('',#9224,#7290,#7291);
#6327=AXIS2_PLACEMENT_3D('',#9230,#7295,#7296);
#6328=AXIS2_PLACEMENT_3D('',#9232,#7297,#7298);
#6329=AXIS2_PLACEMENT_3D('',#9235,#7300,#7301);
#6330=AXIS2_PLACEMENT_3D('',#9236,#7302,#7303);
#6331=AXIS2_PLACEMENT_3D('',#9237,#7304,#7305);
#6332=AXIS2_PLACEMENT_3D('',#9238,#7306,#7307);
#6333=AXIS2_PLACEMENT_3D('',#9239,#7308,#7309);
#6334=AXIS2_PLACEMENT_3D('',#9242,#7311,#7312);
#6335=AXIS2_PLACEMENT_3D('',#9345,#7313,#7314);
#6336=AXIS2_PLACEMENT_3D('',#9346,#7315,#7316);
#6337=AXIS2_PLACEMENT_3D('',#9349,#7318,#7319);
#6338=AXIS2_PLACEMENT_3D('',#9350,#7320,#7321);
#6339=AXIS2_PLACEMENT_3D('',#9354,#7323,#7324);
#6340=AXIS2_PLACEMENT_3D('',#9355,#7325,#7326);
#6341=AXIS2_PLACEMENT_3D('',#9356,#7327,#7328);
#6342=AXIS2_PLACEMENT_3D('',#9358,#7329,#7330);
#6343=AXIS2_PLACEMENT_3D('',#9362,#7333,#7334);
#6344=AXIS2_PLACEMENT_3D('',#9364,#7335,#7336);
#6345=AXIS2_PLACEMENT_3D('',#9366,#7337,#7338);
#6346=AXIS2_PLACEMENT_3D('',#9367,#7339,#7340);
#6347=AXIS2_PLACEMENT_3D('',#9475,#7341,#7342);
#6348=AXIS2_PLACEMENT_3D('',#9476,#7343,#7344);
#6349=AXIS2_PLACEMENT_3D('',#9477,#7345,#7346);
#6350=AXIS2_PLACEMENT_3D('',#9478,#7347,#7348);
#6351=AXIS2_PLACEMENT_3D('',#9479,#7349,#7350);
#6352=AXIS2_PLACEMENT_3D('',#9480,#7351,#7352);
#6353=AXIS2_PLACEMENT_3D('',#9481,#7353,#7354);
#6354=AXIS2_PLACEMENT_3D('',#9482,#7355,#7356);
#6355=AXIS2_PLACEMENT_3D('',#9484,#7357,#7358);
#6356=AXIS2_PLACEMENT_3D('',#9485,#7359,#7360);
#6357=AXIS2_PLACEMENT_3D('',#9486,#7361,#7362);
#6358=AXIS2_PLACEMENT_3D('',#9489,#7364,#7365);
#6359=AXIS2_PLACEMENT_3D('',#9490,#7366,#7367);
#6360=AXIS2_PLACEMENT_3D('',#9491,#7368,#7369);
#6361=AXIS2_PLACEMENT_3D('',#9492,#7370,#7371);
#6362=AXIS2_PLACEMENT_3D('',#9495,#7373,#7374);
#6363=AXIS2_PLACEMENT_3D('',#9496,#7375,#7376);
#6364=AXIS2_PLACEMENT_3D('',#9500,#7379,#7380);
#6365=AXIS2_PLACEMENT_3D('',#9502,#7381,#7382);
#6366=AXIS2_PLACEMENT_3D('',#9505,#7384,#7385);
#6367=AXIS2_PLACEMENT_3D('',#9506,#7386,#7387);
#6368=AXIS2_PLACEMENT_3D('',#9507,#7388,#7389);
#6369=AXIS2_PLACEMENT_3D('',#9508,#7390,#7391);
#6370=AXIS2_PLACEMENT_3D('',#9511,#7393,#7394);
#6371=AXIS2_PLACEMENT_3D('',#9512,#7395,#7396);
#6372=AXIS2_PLACEMENT_3D('',#9513,#7397,#7398);
#6373=AXIS2_PLACEMENT_3D('',#9514,#7399,#7400);
#6374=AXIS2_PLACEMENT_3D('',#9515,#7401,#7402);
#6375=AXIS2_PLACEMENT_3D('',#9516,#7403,#7404);
#6376=AXIS2_PLACEMENT_3D('',#9519,#7406,#7407);
#6377=AXIS2_PLACEMENT_3D('',#9520,#7408,#7409);
#6378=AXIS2_PLACEMENT_3D('',#9523,#7411,#7412);
#6379=AXIS2_PLACEMENT_3D('',#9524,#7413,#7414);
#6380=AXIS2_PLACEMENT_3D('',#9525,#7415,#7416);
#6381=AXIS2_PLACEMENT_3D('',#9526,#7417,#7418);
#6382=AXIS2_PLACEMENT_3D('',#9527,#7419,#7420);
#6383=AXIS2_PLACEMENT_3D('',#9528,#7421,#7422);
#6384=AXIS2_PLACEMENT_3D('',#9529,#7423,#7424);
#6385=AXIS2_PLACEMENT_3D('',#9530,#7425,#7426);
#6386=AXIS2_PLACEMENT_3D('',#9531,#7427,#7428);
#6387=AXIS2_PLACEMENT_3D('',#9533,#7429,#7430);
#6388=AXIS2_PLACEMENT_3D('',#9535,#7432,#7433);
#6389=AXIS2_PLACEMENT_3D('',#9537,#7434,#7435);
#6390=AXIS2_PLACEMENT_3D('',#9538,#7436,#7437);
#6391=AXIS2_PLACEMENT_3D('',#9540,#7438,#7439);
#6392=AXIS2_PLACEMENT_3D('',#9542,#7441,#7442);
#6393=AXIS2_PLACEMENT_3D('',#9544,#7444,#7445);
#6394=AXIS2_PLACEMENT_3D('',#9547,#7446,#7447);
#6395=AXIS2_PLACEMENT_3D('',#9549,#7449,#7450);
#6396=AXIS2_PLACEMENT_3D('',#9550,#7451,#7452);
#6397=AXIS2_PLACEMENT_3D('',#9553,#7453,#7454);
#6398=AXIS2_PLACEMENT_3D('',#9554,#7455,#7456);
#6399=AXIS2_PLACEMENT_3D('',#9558,#7458,#7459);
#6400=AXIS2_PLACEMENT_3D('',#9559,#7460,#7461);
#6401=AXIS2_PLACEMENT_3D('',#9560,#7462,#7463);
#6402=AXIS2_PLACEMENT_3D('',#9561,#7464,#7465);
#6403=AXIS2_PLACEMENT_3D('',#9562,#7466,#7467);
#6404=AXIS2_PLACEMENT_3D('',#9564,#7468,#7469);
#6405=AXIS2_PLACEMENT_3D('',#9577,#7470,#7471);
#6406=AXIS2_PLACEMENT_3D('',#9670,#7472,#7473);
#6407=AXIS2_PLACEMENT_3D('',#9692,#7474,#7475);
#6408=AXIS2_PLACEMENT_3D('',#9777,#7476,#7477);
#6409=AXIS2_PLACEMENT_3D('',#9876,#7478,#7479);
#6410=AXIS2_PLACEMENT_3D('',#9877,#7480,#7481);
#6411=AXIS2_PLACEMENT_3D('',#9878,#7482,#7483);
#6412=AXIS2_PLACEMENT_3D('',#9888,#7488,#7489);
#6413=AXIS2_PLACEMENT_3D('',#9899,#7495,#7496);
#6414=AXIS2_PLACEMENT_3D('',#9900,#7497,#7498);
#6415=AXIS2_PLACEMENT_3D('',#9936,#7501,#7502);
#6416=AXIS2_PLACEMENT_3D('',#9955,#7503,#7504);
#6417=AXIS2_PLACEMENT_3D('',#9956,#7505,#7506);
#6418=AXIS2_PLACEMENT_3D('',#9959,#7508,#7509);
#6419=AXIS2_PLACEMENT_3D('',#9960,#7510,#7511);
#6420=AXIS2_PLACEMENT_3D('',#9962,#7512,#7513);
#6421=AXIS2_PLACEMENT_3D('',#9968,#7516,#7517);
#6422=AXIS2_PLACEMENT_3D('',#9972,#7520,#7521);
#6423=AXIS2_PLACEMENT_3D('',#9973,#7522,#7523);
#6424=AXIS2_PLACEMENT_3D('',#10002,#7531,#7532);
#6425=AXIS2_PLACEMENT_3D('',#10003,#7533,#7534);
#6426=AXIS2_PLACEMENT_3D('',#10058,#7536,#7537);
#6427=AXIS2_PLACEMENT_3D('',#10060,#7538,#7539);
#6428=AXIS2_PLACEMENT_3D('',#10064,#7542,#7543);
#6429=AXIS2_PLACEMENT_3D('',#10065,#7544,#7545);
#6430=AXIS2_PLACEMENT_3D('',#10101,#7553,#7554);
#6431=AXIS2_PLACEMENT_3D('',#10102,#7555,#7556);
#6432=AXIS2_PLACEMENT_3D('',#10103,#7557,#7558);
#6433=AXIS2_PLACEMENT_3D('',#10105,#7559,#7560);
#6434=AXIS2_PLACEMENT_3D('',#10110,#7563,#7564);
#6435=AXIS2_PLACEMENT_3D('',#10111,#7565,#7566);
#6436=AXIS2_PLACEMENT_3D('',#10114,#7567,#7568);
#6437=AXIS2_PLACEMENT_3D('',#10115,#7569,#7570);
#6438=AXIS2_PLACEMENT_3D('',#10116,#7571,#7572);
#6439=AXIS2_PLACEMENT_3D('',#10117,#7573,#7574);
#6440=AXIS2_PLACEMENT_3D('',#10135,#7584,#7585);
#6441=AXIS2_PLACEMENT_3D('',#10137,#7586,#7587);
#6442=AXIS2_PLACEMENT_3D('',#10138,#7588,#7589);
#6443=AXIS2_PLACEMENT_3D('',#10140,#7591,#7592);
#6444=AXIS2_PLACEMENT_3D('',#10141,#7593,#7594);
#6445=AXIS2_PLACEMENT_3D('',#10142,#7595,#7596);
#6446=AXIS2_PLACEMENT_3D('',#10143,#7597,#7598);
#6447=AXIS2_PLACEMENT_3D('',#10145,#7600,#7601);
#6448=AXIS2_PLACEMENT_3D('',#10147,#7603,#7604);
#6449=AXIS2_PLACEMENT_3D('',#10148,#7605,#7606);
#6450=AXIS2_PLACEMENT_3D('',#10150,#7608,#7609);
#6451=AXIS2_PLACEMENT_3D('',#10152,#7611,#7612);
#6452=AXIS2_PLACEMENT_3D('',#10153,#7613,#7614);
#6453=AXIS2_PLACEMENT_3D('',#10154,#7615,#7616);
#6454=AXIS2_PLACEMENT_3D('',#10199,#7617,#7618);
#6455=AXIS2_PLACEMENT_3D('',#10252,#7619,#7620);
#6456=AXIS2_PLACEMENT_3D('',#10253,#7621,#7622);
#6457=AXIS2_PLACEMENT_3D('',#10254,#7623,#7624);
#6458=AXIS2_PLACEMENT_3D('',#10255,#7625,#7626);
#6459=AXIS2_PLACEMENT_3D('',#10256,#7627,#7628);
#6460=AXIS2_PLACEMENT_3D('',#10258,#7629,#7630);
#6461=AXIS2_PLACEMENT_3D('',#10259,#7631,#7632);
#6462=AXIS2_PLACEMENT_3D('',#10260,#7633,#7634);
#6463=AXIS2_PLACEMENT_3D('',#10265,#7637,#7638);
#6464=AXIS2_PLACEMENT_3D('',#10266,#7639,#7640);
#6465=AXIS2_PLACEMENT_3D('',#10268,#7641,#7642);
#6466=AXIS2_PLACEMENT_3D('',#10274,#7646,#7647);
#6467=AXIS2_PLACEMENT_3D('',#10275,#7648,#7649);
#6468=AXIS2_PLACEMENT_3D('',#10277,#7650,#7651);
#6469=AXIS2_PLACEMENT_3D('',#10279,#7653,#7654);
#6470=AXIS2_PLACEMENT_3D('',#10281,#7655,#7656);
#6471=AXIS2_PLACEMENT_3D('',#10284,#7658,#7659);
#6472=AXIS2_PLACEMENT_3D('',#10286,#7660,#7661);
#6473=AXIS2_PLACEMENT_3D('',#10289,#7663,#7664);
#6474=AXIS2_PLACEMENT_3D('',#10291,#7665,#7666);
#6475=AXIS2_PLACEMENT_3D('',#10292,#7667,#7668);
#6476=AXIS2_PLACEMENT_3D('',#10294,#7670,#7671);
#6477=AXIS2_PLACEMENT_3D('',#10295,#7672,#7673);
#6478=AXIS2_PLACEMENT_3D('',#10301,#7677,#7678);
#6479=AXIS2_PLACEMENT_3D('',#10302,#7679,#7680);
#6480=AXIS2_PLACEMENT_3D('',#10303,#7681,#7682);
#6481=AXIS2_PLACEMENT_3D('',#10305,#7683,#7684);
#6482=AXIS2_PLACEMENT_3D('',#10306,#7685,#7686);
#6483=AXIS2_PLACEMENT_3D('',#10307,#7687,#7688);
#6484=AXIS2_PLACEMENT_3D('',#10309,#7690,#7691);
#6485=AXIS2_PLACEMENT_3D('',#10313,#7694,#7695);
#6486=AXIS2_PLACEMENT_3D('',#10314,#7696,#7697);
#6487=AXIS2_PLACEMENT_3D('',#10315,#7698,#7699);
#6488=AXIS2_PLACEMENT_3D('',#10316,#7700,#7701);
#6489=AXIS2_PLACEMENT_3D('',#10317,#7702,#7703);
#6490=AXIS2_PLACEMENT_3D('',#10318,#7704,#7705);
#6491=AXIS2_PLACEMENT_3D('',#10319,#7706,#7707);
#6492=AXIS2_PLACEMENT_3D('',#10320,#7708,#7709);
#6493=AXIS2_PLACEMENT_3D('',#10321,#7710,#7711);
#6494=AXIS2_PLACEMENT_3D('',#10322,#7712,#7713);
#6495=AXIS2_PLACEMENT_3D('',#10324,#7714,#7715);
#6496=AXIS2_PLACEMENT_3D('',#10326,#7717,#7718);
#6497=AXIS2_PLACEMENT_3D('',#10330,#7721,#7722);
#6498=AXIS2_PLACEMENT_3D('',#10331,#7723,#7724);
#6499=AXIS2_PLACEMENT_3D('',#10332,#7725,#7726);
#6500=AXIS2_PLACEMENT_3D('',#10333,#7727,#7728);
#6501=AXIS2_PLACEMENT_3D('',#10334,#7729,#7730);
#6502=AXIS2_PLACEMENT_3D('',#10335,#7731,#7732);
#6503=AXIS2_PLACEMENT_3D('',#10336,#7733,#7734);
#6504=AXIS2_PLACEMENT_3D('',#10337,#7735,#7736);
#6505=AXIS2_PLACEMENT_3D('',#10338,#7737,#7738);
#6506=AXIS2_PLACEMENT_3D('',#10339,#7739,#7740);
#6507=AXIS2_PLACEMENT_3D('',#10340,#7741,#7742);
#6508=AXIS2_PLACEMENT_3D('',#10341,#7743,#7744);
#6509=AXIS2_PLACEMENT_3D('',#10342,#7745,#7746);
#6510=AXIS2_PLACEMENT_3D('',#10343,#7747,#7748);
#6511=AXIS2_PLACEMENT_3D('',#10345,#7750,#7751);
#6512=AXIS2_PLACEMENT_3D('',#10347,#7753,#7754);
#6513=AXIS2_PLACEMENT_3D('',#10348,#7755,#7756);
#6514=AXIS2_PLACEMENT_3D('',#10350,#7757,#7758);
#6515=AXIS2_PLACEMENT_3D('',#10353,#7760,#7761);
#6516=AXIS2_PLACEMENT_3D('',#10354,#7762,#7763);
#6517=AXIS2_PLACEMENT_3D('',#10356,#7764,#7765);
#6518=AXIS2_PLACEMENT_3D('',#10357,#7766,#7767);
#6519=AXIS2_PLACEMENT_3D('',#10359,#7768,#7769);
#6520=AXIS2_PLACEMENT_3D('',#10362,#7771,#7772);
#6521=AXIS2_PLACEMENT_3D('',#10363,#7773,#7774);
#6522=AXIS2_PLACEMENT_3D('',#10365,#7775,#7776);
#7226=DIRECTION('axis',(0.,0.,1.));
#7227=DIRECTION('refdir',(1.,0.,0.));
#7228=DIRECTION('center_axis',(0.,0.,1.));
#7229=DIRECTION('ref_axis',(1.,0.,0.));
#7230=DIRECTION('',(1.,0.,0.));
#7231=DIRECTION('',(0.,-1.,0.));
#7232=DIRECTION('',(-1.,0.,0.));
#7233=DIRECTION('',(-1.,0.,0.));
#7234=DIRECTION('',(0.,1.,0.));
#7235=DIRECTION('center_axis',(0.,0.,1.));
#7236=DIRECTION('ref_axis',(1.,0.,0.));
#7237=DIRECTION('center_axis',(0.,0.,1.));
#7238=DIRECTION('ref_axis',(1.,0.,0.));
#7239=DIRECTION('',(0.,0.,-1.));
#7240=DIRECTION('center_axis',(0.,0.,-1.));
#7241=DIRECTION('ref_axis',(-1.,0.,0.));
#7242=DIRECTION('center_axis',(0.,0.,-1.));
#7243=DIRECTION('ref_axis',(-1.,0.,0.));
#7244=DIRECTION('center_axis',(0.,0.,1.));
#7245=DIRECTION('ref_axis',(-0.998822100792863,-0.0485222729035968,0.));
#7246=DIRECTION('center_axis',(-0.0485222729035999,0.998822100792863,0.));
#7247=DIRECTION('ref_axis',(0.998822100792863,0.0485222729035999,0.));
#7248=DIRECTION('center_axis',(0.,0.,-1.));
#7249=DIRECTION('ref_axis',(-1.,0.,0.));
#7250=DIRECTION('center_axis',(0.,0.,1.));
#7251=DIRECTION('ref_axis',(1.,0.,0.));
#7252=DIRECTION('center_axis',(0.,0.,1.));
#7253=DIRECTION('ref_axis',(1.,0.,0.));
#7254=DIRECTION('center_axis',(0.,0.,1.));
#7255=DIRECTION('ref_axis',(1.,0.,0.));
#7256=DIRECTION('',(0.,0.,1.));
#7257=DIRECTION('center_axis',(0.,0.,1.));
#7258=DIRECTION('ref_axis',(1.,0.,0.));
#7259=DIRECTION('center_axis',(0.,0.,1.));
#7260=DIRECTION('ref_axis',(1.,0.,0.));
#7261=DIRECTION('center_axis',(0.,0.,1.));
#7262=DIRECTION('ref_axis',(-1.,0.,0.));
#7263=DIRECTION('center_axis',(0.,0.,1.));
#7264=DIRECTION('ref_axis',(-0.99941623957466,0.0341640172468879,0.));
#7265=DIRECTION('center_axis',(0.0341640172468871,0.99941623957466,0.));
#7266=DIRECTION('ref_axis',(0.99941623957466,-0.0341640172468871,0.));
#7267=DIRECTION('center_axis',(0.,0.,1.));
#7268=DIRECTION('ref_axis',(-1.,0.,0.));
#7269=DIRECTION('center_axis',(0.,0.,1.));
#7270=DIRECTION('ref_axis',(-1.,0.,0.));
#7271=DIRECTION('center_axis',(0.,0.,1.));
#7272=DIRECTION('ref_axis',(1.,0.,0.));
#7273=DIRECTION('',(0.,0.,-1.));
#7274=DIRECTION('center_axis',(0.,0.,1.));
#7275=DIRECTION('ref_axis',(1.,0.,0.));
#7276=DIRECTION('center_axis',(0.,0.,1.));
#7277=DIRECTION('ref_axis',(1.,0.,0.));
#7278=DIRECTION('',(0.,1.,0.));
#7279=DIRECTION('',(-1.,0.,0.));
#7280=DIRECTION('',(0.,-1.,0.));
#7281=DIRECTION('',(1.,0.,0.));
#7282=DIRECTION('',(1.,0.,0.));
#7283=DIRECTION('center_axis',(0.,1.,0.));
#7284=DIRECTION('ref_axis',(0.,0.,1.));
#7285=DIRECTION('',(0.,1.,0.));
#7286=DIRECTION('center_axis',(0.,1.,0.));
#7287=DIRECTION('ref_axis',(0.,0.,1.));
#7288=DIRECTION('center_axis',(0.,-1.,0.));
#7289=DIRECTION('ref_axis',(1.,0.,0.));
#7290=DIRECTION('center_axis',(1.,0.,0.));
#7291=DIRECTION('ref_axis',(0.,1.,0.));
#7292=DIRECTION('',(0.,0.,-1.));
#7293=DIRECTION('',(0.,-1.,0.));
#7294=DIRECTION('',(0.,0.,-1.));
#7295=DIRECTION('center_axis',(0.,0.,-1.));
#7296=DIRECTION('ref_axis',(1.,0.,0.));
#7297=DIRECTION('center_axis',(0.,0.,1.));
#7298=DIRECTION('ref_axis',(0.,-1.,0.));
#7299=DIRECTION('',(0.,0.,-1.));
#7300=DIRECTION('center_axis',(0.,0.,-1.));
#7301=DIRECTION('ref_axis',(1.,0.,0.));
#7302=DIRECTION('center_axis',(0.707106781186545,0.70710678118655,0.));
#7303=DIRECTION('ref_axis',(0.707106781186545,-0.70710678118655,0.));
#7304=DIRECTION('center_axis',(1.,0.,0.));
#7305=DIRECTION('ref_axis',(0.,-1.,0.));
#7306=DIRECTION('center_axis',(0.,-1.,0.));
#7307=DIRECTION('ref_axis',(0.,0.,-1.));
#7308=DIRECTION('center_axis',(-1.,0.,0.));
#7309=DIRECTION('ref_axis',(0.,0.,-1.));
#7310=DIRECTION('',(-1.,0.,2.676881426896E-11));
#7311=DIRECTION('center_axis',(-0.999999999999956,-2.96157146246387E-7,
0.));
#7312=DIRECTION('ref_axis',(-5.76584526410216E-19,1.94688709598283E-12,
-1.));
#7313=DIRECTION('center_axis',(-1.,0.,0.));
#7314=DIRECTION('ref_axis',(0.,0.,-1.));
#7315=DIRECTION('center_axis',(-1.,0.,0.));
#7316=DIRECTION('ref_axis',(0.,0.,-1.));
#7317=DIRECTION('',(-1.,0.,-2.67704677823E-11));
#7318=DIRECTION('center_axis',(-1.,0.,0.));
#7319=DIRECTION('ref_axis',(0.,0.,-1.));
#7320=DIRECTION('center_axis',(0.,-1.,0.));
#7321=DIRECTION('ref_axis',(1.,0.,0.));
#7322=DIRECTION('',(1.,0.,2.67704677823E-11));
#7323=DIRECTION('center_axis',(0.,-1.,0.));
#7324=DIRECTION('ref_axis',(0.261958162689304,0.,-0.965079230426416));
#7325=DIRECTION('center_axis',(0.,-1.,0.));
#7326=DIRECTION('ref_axis',(0.261958162689304,0.,-0.965079230426416));
#7327=DIRECTION('center_axis',(0.,-1.,0.));
#7328=DIRECTION('ref_axis',(1.,0.,0.));
#7329=DIRECTION('center_axis',(0.,-1.,0.));
#7330=DIRECTION('ref_axis',(-0.261958162689304,0.,0.965079230426416));
#7331=DIRECTION('',(1.,0.,-2.676881426896E-11));
#7332=DIRECTION('',(0.,0.,-1.));
#7333=DIRECTION('center_axis',(0.,1.,0.));
#7334=DIRECTION('ref_axis',(-0.999130476717975,0.,0.0416928110507389));
#7335=DIRECTION('center_axis',(0.0416928110507391,0.,0.999130476717975));
#7336=DIRECTION('ref_axis',(0.999130476717975,0.,-0.0416928110507391));
#7337=DIRECTION('center_axis',(0.,-1.,0.));
#7338=DIRECTION('ref_axis',(-1.,0.,0.));
#7339=DIRECTION('center_axis',(0.,-1.,0.));
#7340=DIRECTION('ref_axis',(-1.,0.,0.));
#7341=DIRECTION('center_axis',(0.999999999999956,-2.96157145634487E-7,0.));
#7342=DIRECTION('ref_axis',(5.76584525218915E-19,1.94688709598283E-12,1.));
#7343=DIRECTION('center_axis',(1.,0.,0.));
#7344=DIRECTION('ref_axis',(0.,0.,1.));
#7345=DIRECTION('center_axis',(1.,0.,0.));
#7346=DIRECTION('ref_axis',(0.,0.,1.));
#7347=DIRECTION('center_axis',(1.,0.,0.));
#7348=DIRECTION('ref_axis',(0.,0.,1.));
#7349=DIRECTION('center_axis',(0.707106781186548,0.,-0.707106781186548));
#7350=DIRECTION('ref_axis',(0.707106781186548,0.,0.707106781186548));
#7351=DIRECTION('center_axis',(1.,0.,0.));
#7352=DIRECTION('ref_axis',(0.,0.,1.));
#7353=DIRECTION('center_axis',(-1.,0.,0.));
#7354=DIRECTION('ref_axis',(0.,-1.,0.));
#7355=DIRECTION('center_axis',(-0.707106781186545,0.70710678118655,0.));
#7356=DIRECTION('ref_axis',(-0.707106781186545,-0.70710678118655,0.));
#7357=DIRECTION('center_axis',(0.,-1.,0.));
#7358=DIRECTION('ref_axis',(0.,0.,1.));
#7359=DIRECTION('center_axis',(0.,0.,1.));
#7360=DIRECTION('ref_axis',(-1.,0.,0.));
#7361=DIRECTION('center_axis',(0.,0.,-1.));
#7362=DIRECTION('ref_axis',(0.,-1.,0.));
#7363=DIRECTION('',(0.,0.,-1.));
#7364=DIRECTION('center_axis',(0.,0.,-1.));
#7365=DIRECTION('ref_axis',(0.,-1.,0.));
#7366=DIRECTION('center_axis',(-0.707106781186548,0.,0.707106781186548));
#7367=DIRECTION('ref_axis',(-0.707106781186548,0.,-0.707106781186548));
#7368=DIRECTION('center_axis',(0.,-1.,0.));
#7369=DIRECTION('ref_axis',(-1.,0.,0.));
#7370=DIRECTION('center_axis',(0.,1.,0.));
#7371=DIRECTION('ref_axis',(0.,0.,-1.));
#7372=DIRECTION('',(0.,1.,0.));
#7373=DIRECTION('center_axis',(0.,1.,0.));
#7374=DIRECTION('ref_axis',(0.,0.,-1.));
#7375=DIRECTION('center_axis',(-1.,0.,0.));
#7376=DIRECTION('ref_axis',(0.,-1.,0.));
#7377=DIRECTION('',(0.,-1.,0.));
#7378=DIRECTION('',(0.,0.,-1.));
#7379=DIRECTION('center_axis',(0.,0.,-1.));
#7380=DIRECTION('ref_axis',(-1.,0.,0.));
#7381=DIRECTION('center_axis',(0.,0.,1.));
#7382=DIRECTION('ref_axis',(0.,1.,0.));
#7383=DIRECTION('',(0.,0.,-1.));
#7384=DIRECTION('center_axis',(0.,0.,-1.));
#7385=DIRECTION('ref_axis',(-1.,0.,0.));
#7386=DIRECTION('center_axis',(-0.707106781186545,-0.70710678118655,0.));
#7387=DIRECTION('ref_axis',(-0.707106781186545,0.70710678118655,0.));
#7388=DIRECTION('center_axis',(-1.,0.,0.));
#7389=DIRECTION('ref_axis',(0.,1.,0.));
#7390=DIRECTION('center_axis',(1.,0.,0.));
#7391=DIRECTION('ref_axis',(0.,0.,-1.));
#7392=DIRECTION('',(1.,0.,0.));
#7393=DIRECTION('center_axis',(1.,0.,0.));
#7394=DIRECTION('ref_axis',(0.,0.,-1.));
#7395=DIRECTION('center_axis',(-0.707106781186545,0.70710678118655,0.));
#7396=DIRECTION('ref_axis',(0.707106781186545,0.70710678118655,0.));
#7397=DIRECTION('center_axis',(0.,1.,0.));
#7398=DIRECTION('ref_axis',(1.,0.,0.));
#7399=DIRECTION('center_axis',(0.,0.,-1.));
#7400=DIRECTION('ref_axis',(0.,1.,0.));
#7401=DIRECTION('center_axis',(0.,-1.,0.));
#7402=DIRECTION('ref_axis',(0.,0.,-1.));
#7403=DIRECTION('center_axis',(0.,0.,-1.));
#7404=DIRECTION('ref_axis',(0.,1.,0.));
#7405=DIRECTION('',(0.,0.,-1.));
#7406=DIRECTION('center_axis',(0.,0.,1.));
#7407=DIRECTION('ref_axis',(1.,0.,0.));
#7408=DIRECTION('center_axis',(0.,1.,0.));
#7409=DIRECTION('ref_axis',(-1.,0.,0.));
#7410=DIRECTION('',(-1.,0.,0.));
#7411=DIRECTION('center_axis',(0.,1.,0.));
#7412=DIRECTION('ref_axis',(1.,0.,0.));
#7413=DIRECTION('center_axis',(-1.,0.,0.));
#7414=DIRECTION('ref_axis',(0.,0.,1.));
#7415=DIRECTION('center_axis',(-1.,0.,0.));
#7416=DIRECTION('ref_axis',(0.,0.,1.));
#7417=DIRECTION('center_axis',(1.,0.,0.));
#7418=DIRECTION('ref_axis',(0.,1.,0.));
#7419=DIRECTION('center_axis',(0.,0.70710678118655,-0.707106781186545));
#7420=DIRECTION('ref_axis',(0.,0.70710678118655,0.707106781186545));
#7421=DIRECTION('center_axis',(-0.707106781186548,0.,-0.707106781186548));
#7422=DIRECTION('ref_axis',(-0.707106781186548,0.,0.707106781186548));
#7423=DIRECTION('center_axis',(0.,1.,0.));
#7424=DIRECTION('ref_axis',(-1.,0.,0.));
#7425=DIRECTION('center_axis',(0.,-1.,0.));
#7426=DIRECTION('ref_axis',(0.,0.,1.));
#7427=DIRECTION('center_axis',(0.,1.,0.));
#7428=DIRECTION('ref_axis',(1.,0.,0.));
#7429=DIRECTION('center_axis',(0.,1.,0.));
#7430=DIRECTION('ref_axis',(1.,0.,0.));
#7431=DIRECTION('',(0.,-1.,0.));
#7432=DIRECTION('center_axis',(0.,1.,0.));
#7433=DIRECTION('ref_axis',(1.,0.,0.));
#7434=DIRECTION('center_axis',(0.,1.,0.));
#7435=DIRECTION('ref_axis',(1.,0.,0.));
#7436=DIRECTION('center_axis',(0.,1.,0.));
#7437=DIRECTION('ref_axis',(1.,0.,0.));
#7438=DIRECTION('center_axis',(0.,1.,0.));
#7439=DIRECTION('ref_axis',(1.,0.,0.));
#7440=DIRECTION('',(-0.707106781186547,0.707106781186548,8.65956056235493E-17));
#7441=DIRECTION('center_axis',(0.,1.,0.));
#7442=DIRECTION('ref_axis',(1.,0.,0.));
#7443=DIRECTION('',(0.,1.,0.));
#7444=DIRECTION('center_axis',(0.,-1.,0.));
#7445=DIRECTION('ref_axis',(-1.,0.,0.));
#7446=DIRECTION('center_axis',(0.,1.,0.));
#7447=DIRECTION('ref_axis',(-1.,0.,0.));
#7448=DIRECTION('',(-0.0697564737441253,0.997564050259824,-8.54270422905495E-18));
#7449=DIRECTION('center_axis',(0.,1.,0.));
#7450=DIRECTION('ref_axis',(-1.,0.,0.));
#7451=DIRECTION('center_axis',(0.,-1.,0.));
#7452=DIRECTION('ref_axis',(-1.,0.,0.));
#7453=DIRECTION('center_axis',(0.,1.,0.));
#7454=DIRECTION('ref_axis',(-1.,0.,0.));
#7455=DIRECTION('center_axis',(0.,1.,0.));
#7456=DIRECTION('ref_axis',(-1.,0.,0.));
#7457=DIRECTION('',(-0.0697564737441253,0.997564050259824,-8.54270422905495E-18));
#7458=DIRECTION('center_axis',(0.,1.,0.));
#7459=DIRECTION('ref_axis',(0.,0.,1.));
#7460=DIRECTION('center_axis',(0.,1.,0.));
#7461=DIRECTION('ref_axis',(0.,0.,1.));
#7462=DIRECTION('center_axis',(0.,1.,0.));
#7463=DIRECTION('ref_axis',(0.,0.,-1.));
#7464=DIRECTION('center_axis',(1.,0.,-1.22464679914735E-16));
#7465=DIRECTION('ref_axis',(1.22464679914735E-16,0.,1.));
#7466=DIRECTION('center_axis',(0.,1.,0.));
#7467=DIRECTION('ref_axis',(-0.00148595964285994,0.,-0.999998895961361));
#7468=DIRECTION('center_axis',(-0.99999889596136,0.,0.00148595964286006));
#7469=DIRECTION('ref_axis',(0.00148595964286006,0.,0.99999889596136));
#7470=DIRECTION('center_axis',(0.,1.,0.));
#7471=DIRECTION('ref_axis',(0.7520613912797,0.,0.659093061522));
#7472=DIRECTION('center_axis',(0.,1.,0.));
#7473=DIRECTION('ref_axis',(0.906252959615387,0.,-0.422735819618294));
#7474=DIRECTION('center_axis',(0.,1.,0.));
#7475=DIRECTION('ref_axis',(-0.7520613912797,0.,-0.659093061522));
#7476=DIRECTION('center_axis',(0.,1.,0.));
#7477=DIRECTION('ref_axis',(-0.906252959678649,0.,0.422735819482676));
#7478=DIRECTION('center_axis',(0.,8.267930667502E-9,-1.));
#7479=DIRECTION('ref_axis',(-1.,1.563194018672E-13,1.29243797662339E-21));
#7480=DIRECTION('center_axis',(0.,0.,-1.));
#7481=DIRECTION('ref_axis',(-1.,0.,0.));
#7482=DIRECTION('center_axis',(-1.,0.,0.));
#7483=DIRECTION('ref_axis',(0.,-1.,0.));
#7484=DIRECTION('',(0.,3.40889233658E-10,-1.));
#7485=DIRECTION('',(-5.132671782924E-14,-2.643911472987E-9,-1.));
#7486=DIRECTION('',(0.,1.,0.));
#7487=DIRECTION('',(0.,-7.255275745268E-12,1.));
#7488=DIRECTION('center_axis',(1.,0.,0.));
#7489=DIRECTION('ref_axis',(0.,1.,0.));
#7490=DIRECTION('',(0.,-1.,0.));
#7491=DIRECTION('',(0.,0.,-1.));
#7492=DIRECTION('',(0.,1.,0.));
#7493=DIRECTION('',(0.,0.,-1.));
#7494=DIRECTION('',(0.,-1.,0.));
#7495=DIRECTION('center_axis',(1.,0.,0.));
#7496=DIRECTION('ref_axis',(0.,0.,-1.));
#7497=DIRECTION('center_axis',(1.,0.,0.));
#7498=DIRECTION('ref_axis',(0.,0.,-1.));
#7499=DIRECTION('',(1.,0.,0.));
#7500=DIRECTION('',(1.,0.,0.));
#7501=DIRECTION('center_axis',(1.,0.,0.));
#7502=DIRECTION('ref_axis',(0.,0.,-1.));
#7503=DIRECTION('center_axis',(1.,0.,0.));
#7504=DIRECTION('ref_axis',(0.,0.,-1.));
#7505=DIRECTION('center_axis',(0.,0.,1.));
#7506=DIRECTION('ref_axis',(1.,0.,0.));
#7507=DIRECTION('',(0.,0.,1.));
#7508=DIRECTION('center_axis',(0.,0.,1.));
#7509=DIRECTION('ref_axis',(1.,0.,0.));
#7510=DIRECTION('center_axis',(0.,0.,1.));
#7511=DIRECTION('ref_axis',(1.,0.,0.));
#7512=DIRECTION('center_axis',(0.,0.,1.));
#7513=DIRECTION('ref_axis',(0.,1.,0.));
#7514=DIRECTION('',(1.,0.,0.));
#7515=DIRECTION('',(0.,1.,0.));
#7516=DIRECTION('center_axis',(0.,0.,1.));
#7517=DIRECTION('ref_axis',(1.,0.,0.));
#7518=DIRECTION('',(-1.,0.,0.));
#7519=DIRECTION('',(-1.,0.,0.));
#7520=DIRECTION('center_axis',(0.,0.,-1.));
#7521=DIRECTION('ref_axis',(1.,0.,0.));
#7522=DIRECTION('center_axis',(0.,0.,1.));
#7523=DIRECTION('ref_axis',(1.,0.,0.));
#7524=DIRECTION('',(0.,1.,0.));
#7525=DIRECTION('',(1.,0.,0.));
#7526=DIRECTION('',(-1.,0.,0.));
#7527=DIRECTION('',(0.,-1.,0.));
#7528=DIRECTION('',(1.,0.,0.));
#7529=DIRECTION('',(0.,1.,0.));
#7530=DIRECTION('',(-1.,0.,0.));
#7531=DIRECTION('center_axis',(0.,0.,1.));
#7532=DIRECTION('ref_axis',(1.,0.,0.));
#7533=DIRECTION('center_axis',(0.,0.,1.));
#7534=DIRECTION('ref_axis',(1.,0.,0.));
#7535=DIRECTION('',(0.,0.,1.));
#7536=DIRECTION('center_axis',(1.,0.,0.));
#7537=DIRECTION('ref_axis',(0.,0.,-1.));
#7538=DIRECTION('center_axis',(1.,0.,0.));
#7539=DIRECTION('ref_axis',(0.,0.,-1.));
#7540=DIRECTION('',(1.,0.,0.));
#7541=DIRECTION('',(1.,0.,0.));
#7542=DIRECTION('center_axis',(1.,0.,0.));
#7543=DIRECTION('ref_axis',(0.,0.,-1.));
#7544=DIRECTION('center_axis',(1.,0.,0.));
#7545=DIRECTION('ref_axis',(0.,1.,0.));
#7546=DIRECTION('',(0.,-3.676570159428E-11,1.));
#7547=DIRECTION('',(0.,-1.,0.));
#7548=DIRECTION('',(0.,0.,-1.));
#7549=DIRECTION('',(2.105217949922E-14,7.33486663786E-9,-1.));
#7550=DIRECTION('',(0.,0.,-1.));
#7551=DIRECTION('',(0.,1.,0.));
#7552=DIRECTION('',(0.,0.,-1.));
#7553=DIRECTION('center_axis',(-1.,0.,0.));
#7554=DIRECTION('ref_axis',(0.,0.866025403784429,0.500000000000017));
#7555=DIRECTION('center_axis',(1.,0.,0.));
#7556=DIRECTION('ref_axis',(0.,0.,-1.));
#7557=DIRECTION('center_axis',(0.,0.,1.));
#7558=DIRECTION('ref_axis',(-1.,0.,0.));
#7559=DIRECTION('center_axis',(0.,0.,-1.));
#7560=DIRECTION('ref_axis',(0.,-1.,0.));
#7561=DIRECTION('',(0.,0.,1.));
#7562=DIRECTION('',(0.,0.,1.));
#7563=DIRECTION('center_axis',(0.,0.,1.));
#7564=DIRECTION('ref_axis',(-1.,0.,0.));
#7565=DIRECTION('center_axis',(0.,0.,1.));
#7566=DIRECTION('ref_axis',(-1.,0.,0.));
#7567=DIRECTION('center_axis',(0.,0.,1.));
#7568=DIRECTION('ref_axis',(-1.,0.,0.));
#7569=DIRECTION('center_axis',(0.,-1.,0.));
#7570=DIRECTION('ref_axis',(0.,0.,-1.));
#7571=DIRECTION('center_axis',(-1.,0.,0.));
#7572=DIRECTION('ref_axis',(0.,1.,0.));
#7573=DIRECTION('center_axis',(0.,0.,1.));
#7574=DIRECTION('ref_axis',(1.,0.,0.));
#7575=DIRECTION('',(0.,1.,0.));
#7576=DIRECTION('',(-1.,0.,0.));
#7577=DIRECTION('',(-1.,0.,0.));
#7578=DIRECTION('',(0.,-1.,0.));
#7579=DIRECTION('',(1.,0.,0.));
#7580=DIRECTION('',(0.,-1.,0.));
#7581=DIRECTION('',(1.,0.,0.));
#7582=DIRECTION('',(0.,1.,0.));
#7583=DIRECTION('',(1.,0.,0.));
#7584=DIRECTION('center_axis',(0.,0.,1.));
#7585=DIRECTION('ref_axis',(0.,-1.,0.));
#7586=DIRECTION('center_axis',(0.,0.,-1.));
#7587=DIRECTION('ref_axis',(1.,0.,0.));
#7588=DIRECTION('center_axis',(0.,0.,1.));
#7589=DIRECTION('ref_axis',(1.,0.,0.));
#7590=DIRECTION('',(0.,0.,1.));
#7591=DIRECTION('center_axis',(0.,1.,0.));
#7592=DIRECTION('ref_axis',(0.,0.,-1.));
#7593=DIRECTION('center_axis',(0.,-1.,0.));
#7594=DIRECTION('ref_axis',(-1.,0.,0.));
#7595=DIRECTION('center_axis',(0.,-0.707106781186546,-0.70710678118655));
#7596=DIRECTION('ref_axis',(0.,0.70710678118655,-0.707106781186545));
#7597=DIRECTION('center_axis',(0.,0.,-1.));
#7598=DIRECTION('ref_axis',(-1.,0.,0.));
#7599=DIRECTION('',(4.284382407013E-8,0.,-0.999999999999999));
#7600=DIRECTION('center_axis',(0.,1.,0.));
#7601=DIRECTION('ref_axis',(-1.,0.,0.));
#7602=DIRECTION('',(-9.69930517813E-9,-3.46741652564E-14,-1.));
#7603=DIRECTION('center_axis',(0.,1.,0.));
#7604=DIRECTION('ref_axis',(-1.,0.,0.));
#7605=DIRECTION('center_axis',(0.,1.,0.));
#7606=DIRECTION('ref_axis',(-1.,0.,0.));
#7607=DIRECTION('',(5.264483512846E-9,0.,-1.));
#7608=DIRECTION('center_axis',(0.,1.,0.));
#7609=DIRECTION('ref_axis',(-1.,0.,0.));
#7610=DIRECTION('',(-1.431997384529E-9,0.,-1.));
#7611=DIRECTION('center_axis',(0.,0.,-1.));
#7612=DIRECTION('ref_axis',(-1.,0.,0.));
#7613=DIRECTION('center_axis',(0.,0.,-1.));
#7614=DIRECTION('ref_axis',(0.,1.,0.));
#7615=DIRECTION('center_axis',(0.,8.975029504145E-9,-1.));
#7616=DIRECTION('ref_axis',(0.,1.,8.975029504145E-9));
#7617=DIRECTION('center_axis',(0.,-2.92549305339806E-6,-0.999999999995721));
#7618=DIRECTION('ref_axis',(0.189648565613596,0.981852036486382,-2.87240131221794E-6));
#7619=DIRECTION('center_axis',(0.,0.,-1.));
#7620=DIRECTION('ref_axis',(0.,1.,0.));
#7621=DIRECTION('center_axis',(0.,0.,-1.));
#7622=DIRECTION('ref_axis',(0.,1.,0.));
#7623=DIRECTION('center_axis',(0.,0.707106781186547,0.707106781186548));
#7624=DIRECTION('ref_axis',(0.,0.707106781186548,-0.707106781186547));
#7625=DIRECTION('center_axis',(0.,-1.,0.));
#7626=DIRECTION('ref_axis',(0.,0.,-1.));
#7627=DIRECTION('center_axis',(0.,0.,1.));
#7628=DIRECTION('ref_axis',(0.,-1.,0.));
#7629=DIRECTION('center_axis',(1.,0.,0.));
#7630=DIRECTION('ref_axis',(0.,0.,-1.));
#7631=DIRECTION('center_axis',(0.,0.,1.));
#7632=DIRECTION('ref_axis',(0.,-1.,0.));
#7633=DIRECTION('center_axis',(0.,0.,1.));
#7634=DIRECTION('ref_axis',(0.,-1.,0.));
#7635=DIRECTION('',(0.,0.,1.));
#7636=DIRECTION('',(0.,0.,1.));
#7637=DIRECTION('center_axis',(0.,0.,-1.));
#7638=DIRECTION('ref_axis',(1.,0.,0.));
#7639=DIRECTION('center_axis',(0.,1.,0.));
#7640=DIRECTION('ref_axis',(-1.,0.,0.));
#7641=DIRECTION('center_axis',(0.,1.,0.));
#7642=DIRECTION('ref_axis',(1.,0.,0.));
#7643=DIRECTION('',(1.,0.,0.));
#7644=DIRECTION('',(0.,0.,-1.));
#7645=DIRECTION('',(-1.,0.,0.));
#7646=DIRECTION('center_axis',(0.,1.,0.));
#7647=DIRECTION('ref_axis',(1.,0.,0.));
#7648=DIRECTION('center_axis',(0.,1.,0.));
#7649=DIRECTION('ref_axis',(1.,0.,0.));
#7650=DIRECTION('center_axis',(0.,1.,0.));
#7651=DIRECTION('ref_axis',(1.,0.,0.));
#7652=DIRECTION('',(0.,1.,0.));
#7653=DIRECTION('center_axis',(0.,-1.,0.));
#7654=DIRECTION('ref_axis',(1.,0.,0.));
#7655=DIRECTION('center_axis',(0.,-1.,0.));
#7656=DIRECTION('ref_axis',(0.,0.,1.));
#7657=DIRECTION('',(0.,0.,1.));
#7658=DIRECTION('center_axis',(0.,-1.,0.));
#7659=DIRECTION('ref_axis',(-1.,0.,0.));
#7660=DIRECTION('center_axis',(0.,-1.,0.));
#7661=DIRECTION('ref_axis',(0.,0.,-1.));
#7662=DIRECTION('',(0.,0.,1.));
#7663=DIRECTION('center_axis',(0.,-1.,0.));
#7664=DIRECTION('ref_axis',(1.,0.,0.));
#7665=DIRECTION('center_axis',(0.,1.,0.));
#7666=DIRECTION('ref_axis',(1.,0.,0.));
#7667=DIRECTION('center_axis',(0.,1.,0.));
#7668=DIRECTION('ref_axis',(1.,0.,0.));
#7669=DIRECTION('',(0.,1.,0.));
#7670=DIRECTION('center_axis',(0.,1.,0.));
#7671=DIRECTION('ref_axis',(1.,0.,0.));
#7672=DIRECTION('center_axis',(0.,1.,0.));
#7673=DIRECTION('ref_axis',(-1.,0.,0.));
#7674=DIRECTION('',(-1.,0.,0.));
#7675=DIRECTION('',(0.,0.,-1.));
#7676=DIRECTION('',(1.,0.,0.));
#7677=DIRECTION('center_axis',(1.,0.,0.));
#7678=DIRECTION('ref_axis',(0.,0.,-1.));
#7679=DIRECTION('center_axis',(1.,0.,0.));
#7680=DIRECTION('ref_axis',(0.,0.,-1.));
#7681=DIRECTION('center_axis',(-0.707106781186547,0.707106781186548,0.));
#7682=DIRECTION('ref_axis',(0.707106781186547,0.707106781186548,0.));
#7683=DIRECTION('center_axis',(0.,1.,0.));
#7684=DIRECTION('ref_axis',(1.,0.,0.));
#7685=DIRECTION('center_axis',(0.,0.,-1.));
#7686=DIRECTION('ref_axis',(0.,1.,0.));
#7687=DIRECTION('center_axis',(0.,-1.,0.));
#7688=DIRECTION('ref_axis',(0.,0.,-1.));
#7689=DIRECTION('',(0.,-1.,0.));
#7690=DIRECTION('center_axis',(1.,0.,0.));
#7691=DIRECTION('ref_axis',(0.,1.,0.));
#7692=DIRECTION('',(0.,1.,0.));
#7693=DIRECTION('',(0.,0.,-1.));
#7694=DIRECTION('center_axis',(0.,1.,0.));
#7695=DIRECTION('ref_axis',(0.,0.,1.));
#7696=DIRECTION('center_axis',(0.,1.,0.));
#7697=DIRECTION('ref_axis',(0.,0.,1.));
#7698=DIRECTION('center_axis',(0.,0.707106781186548,-0.707106781186548));
#7699=DIRECTION('ref_axis',(0.,0.707106781186548,0.707106781186548));
#7700=DIRECTION('center_axis',(1.,0.,0.));
#7701=DIRECTION('ref_axis',(0.,1.,0.));
#7702=DIRECTION('center_axis',(0.,0.,1.));
#7703=DIRECTION('ref_axis',(1.,0.,0.));
#7704=DIRECTION('center_axis',(-1.,0.,0.));
#7705=DIRECTION('ref_axis',(0.,0.,1.));
#7706=DIRECTION('center_axis',(-1.,0.,0.));
#7707=DIRECTION('ref_axis',(0.,0.,1.));
#7708=DIRECTION('center_axis',(-1.,0.,0.));
#7709=DIRECTION('ref_axis',(0.,0.707106781186548,0.707106781186548));
#7710=DIRECTION('center_axis',(0.,0.,-1.));
#7711=DIRECTION('ref_axis',(0.,1.,0.));
#7712=DIRECTION('center_axis',(0.,-1.,0.));
#7713=DIRECTION('ref_axis',(0.,0.,1.));
#7714=DIRECTION('center_axis',(0.,1.,0.));
#7715=DIRECTION('ref_axis',(-1.,0.,0.));
#7716=DIRECTION('',(0.,-1.,0.));
#7717=DIRECTION('center_axis',(-1.,0.,0.));
#7718=DIRECTION('ref_axis',(0.,-1.,0.));
#7719=DIRECTION('',(0.,0.,-1.));
#7720=DIRECTION('',(0.,1.,0.));
#7721=DIRECTION('center_axis',(0.,1.,0.));
#7722=DIRECTION('ref_axis',(0.,0.,-1.));
#7723=DIRECTION('center_axis',(0.,1.,0.));
#7724=DIRECTION('ref_axis',(0.,0.,-1.));
#7725=DIRECTION('center_axis',(-0.707106781186547,-0.707106781186548,0.));
#7726=DIRECTION('ref_axis',(-0.707106781186547,0.707106781186548,0.));
#7727=DIRECTION('center_axis',(0.,0.,-1.));
#7728=DIRECTION('ref_axis',(-1.,0.,0.));
#7729=DIRECTION('center_axis',(-1.,0.,0.));
#7730=DIRECTION('ref_axis',(0.,1.,0.));
#7731=DIRECTION('center_axis',(1.,0.,0.));
#7732=DIRECTION('ref_axis',(0.,0.,-1.));
#7733=DIRECTION('center_axis',(0.,0.,-1.));
#7734=DIRECTION('ref_axis',(-1.,0.,0.));
#7735=DIRECTION('center_axis',(0.,0.,1.));
#7736=DIRECTION('ref_axis',(0.,1.,0.));
#7737=DIRECTION('center_axis',(-0.707106781186547,0.,-0.707106781186548));
#7738=DIRECTION('ref_axis',(-0.707106781186547,0.,0.707106781186548));
#7739=DIRECTION('center_axis',(-1.,0.,0.));
#7740=DIRECTION('ref_axis',(0.,0.,1.));
#7741=DIRECTION('center_axis',(-1.,0.,0.));
#7742=DIRECTION('ref_axis',(0.,0.,1.));
#7743=DIRECTION('center_axis',(1.,0.,0.));
#7744=DIRECTION('ref_axis',(0.,1.,0.));
#7745=DIRECTION('center_axis',(-1.,0.,0.));
#7746=DIRECTION('ref_axis',(0.,0.989089789751212,-0.147313909085001));
#7747=DIRECTION('center_axis',(0.,-1.,0.));
#7748=DIRECTION('ref_axis',(0.,0.,-1.));
#7749=DIRECTION('',(1.,0.,0.));
#7750=DIRECTION('center_axis',(0.,0.,-1.));
#7751=DIRECTION('ref_axis',(0.,1.,0.));
#7752=DIRECTION('',(1.,0.,0.));
#7753=DIRECTION('center_axis',(0.,1.,0.));
#7754=DIRECTION('ref_axis',(0.,0.,1.));
#7755=DIRECTION('center_axis',(-1.,0.,0.));
#7756=DIRECTION('ref_axis',(0.,-1.,0.));
#7757=DIRECTION('center_axis',(-1.,0.,0.));
#7758=DIRECTION('ref_axis',(0.,1.,0.));
#7759=DIRECTION('',(1.,0.,0.));
#7760=DIRECTION('center_axis',(-1.,0.,0.));
#7761=DIRECTION('ref_axis',(0.,1.,0.));
#7762=DIRECTION('center_axis',(-1.,0.,0.));
#7763=DIRECTION('ref_axis',(0.,-1.,0.));
#7764=DIRECTION('center_axis',(1.,0.,0.));
#7765=DIRECTION('ref_axis',(0.,1.,0.));
#7766=DIRECTION('center_axis',(1.,0.,0.));
#7767=DIRECTION('ref_axis',(0.,1.,0.));
#7768=DIRECTION('center_axis',(1.,0.,0.));
#7769=DIRECTION('ref_axis',(0.,-1.,0.));
#7770=DIRECTION('',(-1.,0.,0.));
#7771=DIRECTION('center_axis',(1.,0.,0.));
#7772=DIRECTION('ref_axis',(0.,-1.,0.));
#7773=DIRECTION('center_axis',(1.,0.,0.));
#7774=DIRECTION('ref_axis',(0.,1.,0.));
#7775=DIRECTION('center_axis',(-1.,0.,0.));
#7776=DIRECTION('ref_axis',(0.,-1.,0.));
#9101=CARTESIAN_POINT('',(0.,0.,0.));
#9102=CARTESIAN_POINT('Origin',(0.,0.,-7.));
#9103=CARTESIAN_POINT('',(-7.,116.,-7.));
#9104=CARTESIAN_POINT('',(7.,116.,-7.));
#9105=CARTESIAN_POINT('',(-7.,116.,-7.));
#9106=CARTESIAN_POINT('',(7.,102.,-7.));
#9107=CARTESIAN_POINT('',(7.,116.,-7.));
#9108=CARTESIAN_POINT('',(1.628604434127,101.999999999997,-7.));
#9109=CARTESIAN_POINT('',(7.,102.,-7.));
#9110=CARTESIAN_POINT('',(-1.628621699819,102.,-7.));
#9111=CARTESIAN_POINT('Ctrl Pts',(1.62860443416043,101.999999999993,-7.));
#9112=CARTESIAN_POINT('Ctrl Pts',(1.4853123590287,101.999999921671,-7.));
#9113=CARTESIAN_POINT('Ctrl Pts',(1.21253741465399,101.99898584252,-7.));
#9114=CARTESIAN_POINT('Ctrl Pts',(0.8573044679824,101.9969182521,-7.));
#9115=CARTESIAN_POINT('Ctrl Pts',(0.5185327144029,101.9951338414,-7.));
#9116=CARTESIAN_POINT('Ctrl Pts',(0.1644709951681,101.9940222806,-7.));
#9117=CARTESIAN_POINT('Ctrl Pts',(-0.2218799388119,101.9940840565,-7.));
#9118=CARTESIAN_POINT('Ctrl Pts',(-0.6437910911378,101.9956599723,-7.));
#9119=CARTESIAN_POINT('Ctrl Pts',(-1.107253407488,101.998441137,-7.));
#9120=CARTESIAN_POINT('Ctrl Pts',(-1.449586300965,101.9999999758,-7.));
#9121=CARTESIAN_POINT('Ctrl Pts',(-1.628621699819,102.,-7.));
#9122=CARTESIAN_POINT('',(-7.,102.,-7.));
#9123=CARTESIAN_POINT('',(-1.628621699819,102.,-7.));
#9124=CARTESIAN_POINT('',(-7.,102.,-7.));
#9125=CARTESIAN_POINT('',(-4.5,109.,-7.));
#9126=CARTESIAN_POINT('Origin',(0.,109.,-7.));
#9127=CARTESIAN_POINT('Origin',(0.,109.,-7.));
#9128=CARTESIAN_POINT('',(-4.5,109.,-11.));
#9129=CARTESIAN_POINT('',(-4.5,109.,-7.));
#9130=CARTESIAN_POINT('',(4.49469945356788,109.218350228066,-11.));
#9131=CARTESIAN_POINT('Origin',(0.,109.,-11.));
#9132=CARTESIAN_POINT('Origin',(0.,109.,-11.));
#9133=CARTESIAN_POINT('Origin',(0.,109.,-11.));
#9134=CARTESIAN_POINT('',(3.99528840317145,109.194089091614,-11.5));
#9135=CARTESIAN_POINT('Origin',(3.99528840317145,109.194089091614,-11.));
#9136=CARTESIAN_POINT('Origin',(0.,109.,-11.5));
#9137=CARTESIAN_POINT('Origin',(0.,0.,-11.5));
#9138=CARTESIAN_POINT('',(-2.5,109.,-11.5));
#9139=CARTESIAN_POINT('Origin',(0.,109.,-11.5));
#9140=CARTESIAN_POINT('Origin',(0.,109.,11.5));
#9141=CARTESIAN_POINT('',(-2.5,109.,11.5));
#9142=CARTESIAN_POINT('',(-2.5,109.,11.5));
#9143=CARTESIAN_POINT('Origin',(0.,109.,11.5));
#9144=CARTESIAN_POINT('',(1.25,111.1650635095,0.));
#9145=CARTESIAN_POINT('',(-1.25,111.165063509461,1.53080849893419E-16));
#9146=CARTESIAN_POINT('Ctrl Pts',(1.25,111.165063509461,1.04083408558608E-16));
#9147=CARTESIAN_POINT('Ctrl Pts',(1.25,111.165063509461,-0.160381333700613));
#9148=CARTESIAN_POINT('Ctrl Pts',(1.21735698059595,111.184781794941,-0.32892325157911));
#9149=CARTESIAN_POINT('Ctrl Pts',(1.08903588717028,111.251495015576,-0.635727949384779));
#9150=CARTESIAN_POINT('Ctrl Pts',(0.993444785163793,111.297125584436,-0.774322167802576));
#9151=CARTESIAN_POINT('Ctrl Pts',(0.774620837257829,111.379833262588,-0.993146115708541));
#9152=CARTESIAN_POINT('Ctrl Pts',(0.635925947642968,111.422831051299,-1.08895634990573));
#9153=CARTESIAN_POINT('Ctrl Pts',(0.328681344361066,111.483239960438,-1.21745488233641));
#9154=CARTESIAN_POINT('Ctrl Pts',(0.159944126385861,111.5,-1.25));
#9155=CARTESIAN_POINT('Ctrl Pts',(-0.159944126385861,111.5,-1.25));
#9156=CARTESIAN_POINT('Ctrl Pts',(-0.328681344361067,111.483239960438,-1.21745488233641));
#9157=CARTESIAN_POINT('Ctrl Pts',(-0.635925947642968,111.422831051299,-1.08895634990573));
#9158=CARTESIAN_POINT('Ctrl Pts',(-0.774620837257829,111.379833262588,-0.993146115708541));
#9159=CARTESIAN_POINT('Ctrl Pts',(-0.993444785163793,111.297125584436,-0.774322167802577));
#9160=CARTESIAN_POINT('Ctrl Pts',(-1.08903588717028,111.251495015576,-0.63572794938478));
#9161=CARTESIAN_POINT('Ctrl Pts',(-1.21735698059595,111.184781794941,-0.328923251579112));
#9162=CARTESIAN_POINT('Ctrl Pts',(-1.25,111.165063509461,-0.160381333700614));
#9163=CARTESIAN_POINT('Ctrl Pts',(-1.25,111.165063509461,-3.46944695195361E-16));
#9164=CARTESIAN_POINT('Ctrl Pts',(-1.25,111.165063509461,2.77555756156289E-16));
#9165=CARTESIAN_POINT('Ctrl Pts',(-1.25,111.165063509461,0.160381333700614));
#9166=CARTESIAN_POINT('Ctrl Pts',(-1.21735698059595,111.184781794941,0.328923251579112));
#9167=CARTESIAN_POINT('Ctrl Pts',(-1.08903588717028,111.251495015576,0.63572794938478));
#9168=CARTESIAN_POINT('Ctrl Pts',(-0.993444785163793,111.297125584436,0.774322167802577));
#9169=CARTESIAN_POINT('Ctrl Pts',(-0.774620837257829,111.379833262588,0.993146115708541));
#9170=CARTESIAN_POINT('Ctrl Pts',(-0.635925947642968,111.422831051299,1.08895634990573));
#9171=CARTESIAN_POINT('Ctrl Pts',(-0.328681344361067,111.483239960438,1.21745488233641));
#9172=CARTESIAN_POINT('Ctrl Pts',(-0.159944126385861,111.5,1.25));
#9173=CARTESIAN_POINT('Ctrl Pts',(0.159944126385861,111.5,1.25));
#9174=CARTESIAN_POINT('Ctrl Pts',(0.328681344361067,111.483239960438,1.21745488233641));
#9175=CARTESIAN_POINT('Ctrl Pts',(0.635925947642968,111.422831051299,1.08895634990573));
#9176=CARTESIAN_POINT('Ctrl Pts',(0.774620837257829,111.379833262588,0.993146115708541));
#9177=CARTESIAN_POINT('Ctrl Pts',(0.993444785163793,111.297125584436,0.774322167802577));
#9178=CARTESIAN_POINT('Ctrl Pts',(1.08903588717028,111.251495015576,0.635727949384779));
#9179=CARTESIAN_POINT('Ctrl Pts',(1.21735698059595,111.184781794941,0.32892325157911));
#9180=CARTESIAN_POINT('Ctrl Pts',(1.25,111.165063509461,0.160381333700614));
#9181=CARTESIAN_POINT('Ctrl Pts',(1.25,111.165063509461,4.33680868994202E-16));
#9182=CARTESIAN_POINT('Origin',(0.,0.,11.5));
#9183=CARTESIAN_POINT('',(3.99766495829864,108.863343931012,11.5));
#9184=CARTESIAN_POINT('Origin',(0.,109.,11.5));
#9185=CARTESIAN_POINT('Origin',(0.,109.,11.));
#9186=CARTESIAN_POINT('',(4.49737307808597,108.846261922389,11.));
#9187=CARTESIAN_POINT('Origin',(3.99766495829864,108.863343931012,11.));
#9188=CARTESIAN_POINT('',(-4.5,109.,11.));
#9189=CARTESIAN_POINT('Origin',(0.,109.,11.));
#9190=CARTESIAN_POINT('Origin',(0.,109.,11.));
#9191=CARTESIAN_POINT('Origin',(0.,109.,7.));
#9192=CARTESIAN_POINT('',(-4.5,109.,7.));
#9193=CARTESIAN_POINT('',(-4.5,109.,7.));
#9194=CARTESIAN_POINT('Origin',(0.,109.,7.));
#9195=CARTESIAN_POINT('Origin',(0.,0.,7.));
#9196=CARTESIAN_POINT('',(7.,102.,7.));
#9197=CARTESIAN_POINT('',(7.,116.,7.));
#9198=CARTESIAN_POINT('',(7.,102.,7.));
#9199=CARTESIAN_POINT('',(-7.,116.,7.));
#9200=CARTESIAN_POINT('',(7.,116.,7.));
#9201=CARTESIAN_POINT('',(-7.,102.,7.));
#9202=CARTESIAN_POINT('',(-7.,116.,7.));
#9203=CARTESIAN_POINT('',(-1.628604434127,101.999999999997,7.));
#9204=CARTESIAN_POINT('',(-7.,102.,7.));
#9205=CARTESIAN_POINT('',(1.628621699819,102.,7.));
#9206=CARTESIAN_POINT('Ctrl Pts',(-1.62860443416043,101.999999999993,7.));
#9207=CARTESIAN_POINT('Ctrl Pts',(-1.4853123590287,101.999999921671,7.));
#9208=CARTESIAN_POINT('Ctrl Pts',(-1.21253741465399,101.99898584252,7.));
#9209=CARTESIAN_POINT('Ctrl Pts',(-0.8573044679823,101.9969182521,7.));
#9210=CARTESIAN_POINT('Ctrl Pts',(-0.5185327144029,101.9951338414,7.));
#9211=CARTESIAN_POINT('Ctrl Pts',(-0.1644709951681,101.9940222806,7.));
#9212=CARTESIAN_POINT('Ctrl Pts',(0.2218799388119,101.9940840565,7.));
#9213=CARTESIAN_POINT('Ctrl Pts',(0.6437910911378,101.9956599723,7.));
#9214=CARTESIAN_POINT('Ctrl Pts',(1.107253407488,101.998441137,7.));
#9215=CARTESIAN_POINT('Ctrl Pts',(1.449586300965,101.9999999758,7.));
#9216=CARTESIAN_POINT('Ctrl Pts',(1.628621699819,102.,7.));
#9217=CARTESIAN_POINT('',(1.628621699819,102.,7.));
#9218=CARTESIAN_POINT('Origin',(7.,-143.7058229487,6.));
#9219=CARTESIAN_POINT('',(8.,102.,6.));
#9220=CARTESIAN_POINT('',(8.,116.,6.));
#9221=CARTESIAN_POINT('',(8.,102.,6.));
#9222=CARTESIAN_POINT('Origin',(7.,116.,6.));
#9223=CARTESIAN_POINT('Origin',(7.,102.,6.));
#9224=CARTESIAN_POINT('Origin',(8.,101.,-7.));
#9225=CARTESIAN_POINT('',(8.,102.,-6.));
#9226=CARTESIAN_POINT('',(8.,102.,6.));
#9227=CARTESIAN_POINT('',(8.,116.,-6.));
#9228=CARTESIAN_POINT('',(8.,116.,-6.));
#9229=CARTESIAN_POINT('',(8.,116.,6.));
#9230=CARTESIAN_POINT('Origin',(7.,102.,43.78380184031));
#9231=CARTESIAN_POINT('',(7.,101.,6.));
#9232=CARTESIAN_POINT('Origin',(7.,102.,6.));
#9233=CARTESIAN_POINT('',(7.,101.,-6.));
#9234=CARTESIAN_POINT('',(7.,101.,6.));
#9235=CARTESIAN_POINT('Origin',(7.,102.,-6.));
#9236=CARTESIAN_POINT('Origin',(7.,102.,-6.));
#9237=CARTESIAN_POINT('Origin',(7.,102.,-6.));
#9238=CARTESIAN_POINT('Origin',(7.,102.,-6.));
#9239=CARTESIAN_POINT('Origin',(75.7512,102.,-6.));
#9240=CARTESIAN_POINT('',(1.62860689419666,100.999999999996,-6.00000151345914));
#9241=CARTESIAN_POINT('',(7.,101.,-6.));
#9242=CARTESIAN_POINT('Origin',(1.628604434127,102.,-6.));
#9243=CARTESIAN_POINT('Ctrl Pts',(1.689481893123,102.1196847108,-6.992808061201));
#9244=CARTESIAN_POINT('Ctrl Pts',(1.669187233917,102.1197065598,-6.992808061201));
#9245=CARTESIAN_POINT('Ctrl Pts',(1.512636201126,102.1197869626,-6.992808061201));
#9246=CARTESIAN_POINT('Ctrl Pts',(1.23556503978,102.1188276871,-6.992808061201));
#9247=CARTESIAN_POINT('Ctrl Pts',(0.8648101546223,102.1166806136,-6.992808061201));
#9248=CARTESIAN_POINT('Ctrl Pts',(0.5109811635092,102.1148120947,-6.992808061201));
#9249=CARTESIAN_POINT('Ctrl Pts',(0.1488522802808,102.1137128273,-6.992808061201));
#9250=CARTESIAN_POINT('Ctrl Pts',(-0.2394130054686,102.1138378158,-6.992808061201));
#9251=CARTESIAN_POINT('Ctrl Pts',(-0.663639050088,102.1154833678,-6.992808061201));
#9252=CARTESIAN_POINT('Ctrl Pts',(-1.130096203131,102.1183003163,-6.992808061201));
#9253=CARTESIAN_POINT('Ctrl Pts',(-1.477116016106,102.1198046106,-6.992808061201));
#9254=CARTESIAN_POINT('Ctrl Pts',(-1.669209716084,102.1197066226,-6.992808061201));
#9255=CARTESIAN_POINT('Ctrl Pts',(-1.689515664192,102.1196849348,-6.992808061201));
#9256=CARTESIAN_POINT('Ctrl Pts',(1.688715228218,101.4207068678,-7.077093790264));
#9257=CARTESIAN_POINT('Ctrl Pts',(1.668689128932,101.4207284853,-7.077093790264));
#9258=CARTESIAN_POINT('Ctrl Pts',(1.514109227167,101.4208080916,-7.077093790264));
#9259=CARTESIAN_POINT('Ctrl Pts',(1.239188923109,101.4198586149,-7.077093790264));
#9260=CARTESIAN_POINT('Ctrl Pts',(0.8689370512759,101.41771466,-7.077093790264));
#9261=CARTESIAN_POINT('Ctrl Pts',(0.5140416525734,101.4158400361,-7.077093790264));
#9262=CARTESIAN_POINT('Ctrl Pts',(0.1498433242845,101.4147339759,-7.077093790264));
#9263=CARTESIAN_POINT('Ctrl Pts',(-0.2409905058727,101.4148598525,-7.077093790264));
#9264=CARTESIAN_POINT('Ctrl Pts',(-0.667428084141,101.4165149357,-7.077093790264));
#9265=CARTESIAN_POINT('Ctrl Pts',(-1.134325060388,101.4193353122,-7.077093790264));
#9266=CARTESIAN_POINT('Ctrl Pts',(-1.479036591025,101.4208256727,-7.077093790264));
#9267=CARTESIAN_POINT('Ctrl Pts',(-1.668711295896,101.4207285315,-7.077093790264));
#9268=CARTESIAN_POINT('Ctrl Pts',(-1.688748453112,101.4207070467,-7.077093790264));
#9269=CARTESIAN_POINT('Ctrl Pts',(1.68816918717,100.9228745154,-6.579261201271));
#9270=CARTESIAN_POINT('Ctrl Pts',(1.668334364073,100.922895968,-6.579261201271));
#9271=CARTESIAN_POINT('Ctrl Pts',(1.515158359163,100.9229750071,-6.579261201271));
#9272=CARTESIAN_POINT('Ctrl Pts',(1.241769958231,100.9220325094,-6.579261201271));
#9273=CARTESIAN_POINT('Ctrl Pts',(0.8718763471198,100.9198907756,-6.579261201271));
#9274=CARTESIAN_POINT('Ctrl Pts',(0.5162214219116,100.9180118035,-6.579261201271));
#9275=CARTESIAN_POINT('Ctrl Pts',(0.1505491746524,100.9169009054,-6.579261201271));
#9276=CARTESIAN_POINT('Ctrl Pts',(-0.2421140475483,100.9170274144,-6.579261201271));
#9277=CARTESIAN_POINT('Ctrl Pts',(-0.6701267444128,100.918689286,-6.579261201271));
#9278=CARTESIAN_POINT('Ctrl Pts',(-1.137336975539,100.9215121041,-6.579261201271));
#9279=CARTESIAN_POINT('Ctrl Pts',(-1.480404480349,100.9229925405,-6.579261201271));
#9280=CARTESIAN_POINT('Ctrl Pts',(-1.668356306539,100.9228960023,-6.579261201271));
#9281=CARTESIAN_POINT('Ctrl Pts',(-1.688202023064,100.9228746621,-6.579261201271));
#9282=CARTESIAN_POINT('Ctrl Pts',(1.688261634851,101.0071602049,-5.880283026469));
#9283=CARTESIAN_POINT('Ctrl Pts',(1.668394427668,101.0071816854,-5.880283026469));
#9284=CARTESIAN_POINT('Ctrl Pts',(1.514980735485,101.0072608205,-5.880283026469));
#9285=CARTESIAN_POINT('Ctrl Pts',(1.241332975131,101.0063171412,-5.880283026469));
#9286=CARTESIAN_POINT('Ctrl Pts',(0.8713787085563,101.0041750314,-5.880283026469));
#9287=CARTESIAN_POINT('Ctrl Pts',(0.5158523752623,101.0022967954,-5.880283026469));
#9288=CARTESIAN_POINT('Ctrl Pts',(0.1504296703963,101.0011867164,-5.880283026469));
#9289=CARTESIAN_POINT('Ctrl Pts',(-0.2419238259118,101.0013131184,-5.880283026469));
#9290=CARTESIAN_POINT('Ctrl Pts',(-0.6696698467433,101.0029738406,-5.880283026469));
#9291=CARTESIAN_POINT('Ctrl Pts',(-1.136827042137,101.0057962454,-5.880283026469));
#9292=CARTESIAN_POINT('Ctrl Pts',(-1.480172889344,101.007278362,-5.880283026469));
#9293=CARTESIAN_POINT('Ctrl Pts',(-1.668416408143,101.0071817217,-5.880283026469));
#9294=CARTESIAN_POINT('Ctrl Pts',(-1.688294536604,101.007160357,-5.880283026469));
#9295=CARTESIAN_POINT('',(-1.62862169826789,100.999999999995,-5.99999999986848));
#9296=CARTESIAN_POINT('Ctrl Pts',(1.62860685825195,100.999999999983,-6.0000009545634));
#9297=CARTESIAN_POINT('Ctrl Pts',(1.52373488016319,100.99999997304,-6.00674566973353));
#9298=CARTESIAN_POINT('Ctrl Pts',(1.42263846185517,100.99978700057,-6.01267762823953));
#9299=CARTESIAN_POINT('Ctrl Pts',(1.32582463231981,100.999497837555,-6.01787098237482));
#9300=CARTESIAN_POINT('Ctrl Pts',(1.29209674790815,100.999397099295,-6.01968023678428));
#9301=CARTESIAN_POINT('Ctrl Pts',(1.25888843888297,100.999286698235,-6.02139992825534));
#9302=CARTESIAN_POINT('Ctrl Pts',(1.22622051364658,100.999171092663,-6.02303342418429));
#9303=CARTESIAN_POINT('Ctrl Pts',(1.13537596273316,100.998849611083,-6.02757592888917));
#9304=CARTESIAN_POINT('Ctrl Pts',(1.04870946239408,100.998489638665,-6.03145127898147));
#9305=CARTESIAN_POINT('Ctrl Pts',(0.964146579740458,100.998135827758,-6.03481770912858));
#9306=CARTESIAN_POINT('Ctrl Pts',(0.931009084803032,100.997997180556,-6.03613690566559));
#9307=CARTESIAN_POINT('Ctrl Pts',(0.898194045077884,100.997859230698,-6.03737801560314));
#9308=CARTESIAN_POINT('Ctrl Pts',(0.865574716854578,100.997724090006,-6.03855077139743));
#9309=CARTESIAN_POINT('Ctrl Pts',(0.763673785219037,100.997301918145,-6.04221439399569));
#9310=CARTESIAN_POINT('Ctrl Pts',(0.663692099762057,100.996905553624,-6.04521010595944));
#9311=CARTESIAN_POINT('Ctrl Pts',(0.562039110946944,100.996569111419,-6.04760859093508));
#9312=CARTESIAN_POINT('Ctrl Pts',(0.548114095188321,100.996523023615,-6.04793714931268));
#9313=CARTESIAN_POINT('Ctrl Pts',(0.534157650522232,100.996478102747,-6.04825450644789));
#9314=CARTESIAN_POINT('Ctrl Pts',(0.520160493462915,100.996434487254,-6.04856084923628));
#9315=CARTESIAN_POINT('Ctrl Pts',(0.412198444871786,100.996098074806,-6.05092371441429));
#9316=CARTESIAN_POINT('Ctrl Pts',(0.301819293815625,100.995835695599,-6.0526309202976));
#9317=CARTESIAN_POINT('Ctrl Pts',(0.186840756394499,100.995693614002,-6.05353748689817));
#9318=CARTESIAN_POINT('Ctrl Pts',(0.178092147645217,100.995682803147,-6.05360646669798));
#9319=CARTESIAN_POINT('Ctrl Pts',(0.169316919910494,100.995672713175,-6.05367081239838));
#9320=CARTESIAN_POINT('Ctrl Pts',(0.160514117704065,100.995663377513,-6.05373046080016));
#9321=CARTESIAN_POINT('Ctrl Pts',(0.0496839098288051,100.995545838423,-6.05448145401959));
#9322=CARTESIAN_POINT('Ctrl Pts',(-0.0655181192494277,100.995546458708,
-6.05448756792474));
#9323=CARTESIAN_POINT('Ctrl Pts',(-0.185310647992566,100.995691809128,-6.05354829979092));
#9324=CARTESIAN_POINT('Ctrl Pts',(-0.200078909707018,100.995709728218,-6.05343250494323));
#9325=CARTESIAN_POINT('Ctrl Pts',(-0.214916879107109,100.995729871175,-6.05330234750083));
#9326=CARTESIAN_POINT('Ctrl Pts',(-0.229824912171414,100.995752309851,-6.05315745718398));
#9327=CARTESIAN_POINT('Ctrl Pts',(-0.340529448807116,100.995918935677,-6.05208152615263));
#9328=CARTESIAN_POINT('Ctrl Pts',(-0.455099630540629,100.996212269576,-6.0501929592695));
#9329=CARTESIAN_POINT('Ctrl Pts',(-0.573986781723262,100.996609420841,-6.04732336142487));
#9330=CARTESIAN_POINT('Ctrl Pts',(-0.600974002364567,100.996699573634,-6.0466719666407));
#9331=CARTESIAN_POINT('Ctrl Pts',(-0.628183462748757,100.996795071311,-6.04597004841208));
#9332=CARTESIAN_POINT('Ctrl Pts',(-0.655620049589773,100.996895635329,-6.04521569132264));
#9333=CARTESIAN_POINT('Ctrl Pts',(-0.764243748505043,100.997293776528,-6.04222912969847));
#9334=CARTESIAN_POINT('Ctrl Pts',(-0.87642962165337,100.997773482976,-6.0384203844328));
#9335=CARTESIAN_POINT('Ctrl Pts',(-0.99232222130473,100.998254098085,-6.0336721558827));
#9336=CARTESIAN_POINT('Ctrl Pts',(-1.03465714845761,100.998429664132,-6.03193765419426));
#9337=CARTESIAN_POINT('Ctrl Pts',(-1.07748630376386,100.998605095003,-6.03007786532948));
#9338=CARTESIAN_POINT('Ctrl Pts',(-1.1208152583269,100.998775489421,-6.02808737922741));
#9339=CARTESIAN_POINT('Ctrl Pts',(-1.22117671474146,100.999170168501,-6.02347688063145));
#9340=CARTESIAN_POINT('Ctrl Pts',(-1.32422004237134,100.999540506896,-6.01816518674119));
#9341=CARTESIAN_POINT('Ctrl Pts',(-1.43019217801676,100.999770783872,-6.01208235725501));
#9342=CARTESIAN_POINT('Ctrl Pts',(-1.49521612659923,100.999912080621,-6.00834996487341));
#9343=CARTESIAN_POINT('Ctrl Pts',(-1.56134223689861,101.00000001874,-6.00432736857725));
#9344=CARTESIAN_POINT('Ctrl Pts',(-1.628621697537,100.999999999981,-5.999999999856));
#9345=CARTESIAN_POINT('Origin',(-1.628621700447,102.,-6.));
#9346=CARTESIAN_POINT('Origin',(8.147852,102.,-6.));
#9347=CARTESIAN_POINT('',(-7.,101.,-6.));
#9348=CARTESIAN_POINT('',(-1.628621697537,101.,-5.999999999856));
#9349=CARTESIAN_POINT('Origin',(-7.,102.,-6.));
#9350=CARTESIAN_POINT('Origin',(-8.,101.,-7.));
#9351=CARTESIAN_POINT('',(1.62862169826789,101.,5.99999999986848));
#9352=CARTESIAN_POINT('',(1.628621697537,101.,5.999999999856));
#9353=CARTESIAN_POINT('',(6.21170021154708,101.,-0.259208631163567));
#9354=CARTESIAN_POINT('Origin',(0.,101.,0.));
#9355=CARTESIAN_POINT('Origin',(0.,101.,0.));
#9356=CARTESIAN_POINT('Origin',(-8.,101.,-7.));
#9357=CARTESIAN_POINT('',(-1.62860689419665,101.,6.00000151345915));
#9358=CARTESIAN_POINT('Origin',(0.,101.,0.));
#9359=CARTESIAN_POINT('',(-7.,101.,6.));
#9360=CARTESIAN_POINT('',(-7.,101.,6.));
#9361=CARTESIAN_POINT('',(-7.,101.,6.));
#9362=CARTESIAN_POINT('Origin',(0.,98.,0.));
#9363=CARTESIAN_POINT('',(3.22161027626912,97.79073057877,-0.134434882788108));
#9364=CARTESIAN_POINT('Origin',(6.21170021154708,98.,-0.259208631163567));
#9365=CARTESIAN_POINT('',(3.22441397929396,97.7907305787699,3.94876825886832E-16));
#9366=CARTESIAN_POINT('Origin',(0.,97.79073057877,0.));
#9367=CARTESIAN_POINT('Origin',(0.,97.79073057877,0.));
#9368=CARTESIAN_POINT('Ctrl Pts',(-1.62860685825194,100.999999999999,6.00000095456346));
#9369=CARTESIAN_POINT('Ctrl Pts',(-1.5402385437957,100.999999982535,6.00568425715639));
#9370=CARTESIAN_POINT('Ctrl Pts',(-1.45455562762397,100.999846865067,6.01079408210886));
#9371=CARTESIAN_POINT('Ctrl Pts',(-1.3718508879526,100.999627223085,6.01536640130176));
#9372=CARTESIAN_POINT('Ctrl Pts',(-1.32221134199258,100.99949539354,6.01811071619376));
#9373=CARTESIAN_POINT('Ctrl Pts',(-1.27364518931805,100.999338908544,6.02066204596849));
#9374=CARTESIAN_POINT('Ctrl Pts',(-1.22622051364658,100.999171092663,6.02303342418429));
#9375=CARTESIAN_POINT('Ctrl Pts',(-1.17181301863647,100.998978567536,6.02575396463326));
#9376=CARTESIAN_POINT('Ctrl Pts',(-1.11890846799787,100.998770692355,6.02821724570366));
#9377=CARTESIAN_POINT('Ctrl Pts',(-1.06705384911434,100.998560015031,6.03048981059644));
#9378=CARTESIAN_POINT('Ctrl Pts',(-1.01372995415689,100.998343368265,6.03282676753944));
#9379=CARTESIAN_POINT('Ctrl Pts',(-0.961516257209871,100.998123681242,6.03496189854049));
#9380=CARTESIAN_POINT('Ctrl Pts',(-0.909929062859923,100.997908538361,6.03691381376813));
#9381=CARTESIAN_POINT('Ctrl Pts',(-0.895096211312916,100.997846678389,6.037475047407));
#9382=CARTESIAN_POINT('Ctrl Pts',(-0.880315213774708,100.99778516074,6.0380208093818));
#9383=CARTESIAN_POINT('Ctrl Pts',(-0.865574716854661,100.997724089988,6.03855077139813));
#9384=CARTESIAN_POINT('Ctrl Pts',(-0.812672184995172,100.997504911662,6.04045276511006));
#9385=CARTESIAN_POINT('Ctrl Pts',(-0.760288018369843,100.997291776737,6.04215834916175));
#9386=CARTESIAN_POINT('Ctrl Pts',(-0.707917910975415,100.997091119445,6.0437082383946));
#9387=CARTESIAN_POINT('Ctrl Pts',(-0.655517128523072,100.996890344621,6.04525903545339));
#9388=CARTESIAN_POINT('Ctrl Pts',(-0.603130360414094,100.996702033618,6.04665393791658));
#9389=CARTESIAN_POINT('Ctrl Pts',(-0.550254983870303,100.996530278855,6.0478819218511));
#9390=CARTESIAN_POINT('Ctrl Pts',(-0.540242132749313,100.996497754172,6.04811446147765));
#9391=CARTESIAN_POINT('Ctrl Pts',(-0.530211769198876,100.996465817122,6.04834086581166));
#9392=CARTESIAN_POINT('Ctrl Pts',(-0.52016049346279,100.996434487268,6.04856084923561));
#9393=CARTESIAN_POINT('Ctrl Pts',(-0.4591600625234,100.996244348761,6.04989591196922));
#9394=CARTESIAN_POINT('Ctrl Pts',(-0.397386423926234,100.996077279975,6.0510104023759));
#9395=CARTESIAN_POINT('Ctrl Pts',(-0.334449136934581,100.995942794773,6.05190134814301));
#9396=CARTESIAN_POINT('Ctrl Pts',(-0.277520856446568,100.995821149692,6.05270722988584));
#9397=CARTESIAN_POINT('Ctrl Pts',(-0.219640398858692,100.995726175995,6.05332981198369));
#9398=CARTESIAN_POINT('Ctrl Pts',(-0.160514117704047,100.995663377514,6.05373046080009));
#9399=CARTESIAN_POINT('Ctrl Pts',(-0.0750025005669668,100.995572554963,
6.05430990072977));
#9400=CARTESIAN_POINT('Ctrl Pts',(0.0131158896791447,100.995550802574,6.05444281080532));
#9401=CARTESIAN_POINT('Ctrl Pts',(0.103931307124153,100.995613638244,6.05404463879305));
#9402=CARTESIAN_POINT('Ctrl Pts',(0.14533109622264,100.995642282978,6.05386312514926));
#9403=CARTESIAN_POINT('Ctrl Pts',(0.187291892296204,100.99568835001,6.05357083005548));
#9404=CARTESIAN_POINT('Ctrl Pts',(0.229824912171415,100.995752309851,6.053157457184));
#9405=CARTESIAN_POINT('Ctrl Pts',(0.311291713085964,100.995874817108,6.05236569197374));
#9406=CARTESIAN_POINT('Ctrl Pts',(0.394857584369436,100.996063677148,6.05112790481686));
#9407=CARTESIAN_POINT('Ctrl Pts',(0.480689955873217,100.996315037781,6.0493902677801));
#9408=CARTESIAN_POINT('Ctrl Pts',(0.537970868394036,100.996482785289,6.04823064194953));
#9409=CARTESIAN_POINT('Ctrl Pts',(0.59626182469888,100.996678124709,6.04684771747587));
#9410=CARTESIAN_POINT('Ctrl Pts',(0.655620049589673,100.996895635349,6.04521569132172));
#9411=CARTESIAN_POINT('Ctrl Pts',(0.743812153458893,100.997218804058,6.04279089138255));
#9412=CARTESIAN_POINT('Ctrl Pts',(0.834359954557442,100.997592544038,6.03982029829353));
#9413=CARTESIAN_POINT('Ctrl Pts',(0.927324292569222,100.997981133951,6.0362495538679));
#9414=CARTESIAN_POINT('Ctrl Pts',(0.990688253627786,100.998245994613,6.03381575489106));
#9415=CARTESIAN_POINT('Ctrl Pts',(1.05517562490491,100.998517286263,6.03110279618582));
#9416=CARTESIAN_POINT('Ctrl Pts',(1.12081525832687,100.998775489428,6.02808737922721));
#9417=CARTESIAN_POINT('Ctrl Pts',(1.20525737992653,100.999107654949,6.02420819538326));
#9418=CARTESIAN_POINT('Ctrl Pts',(1.29160708145152,100.999419290475,6.01982506746926));
#9419=CARTESIAN_POINT('Ctrl Pts',(1.37999323522187,100.999648545207,6.01491167471667));
#9420=CARTESIAN_POINT('Ctrl Pts',(1.46111364923389,100.999858954168,6.01040218496865));
#9421=CARTESIAN_POINT('Ctrl Pts',(1.54394986559642,101.,6.00544603395953));
#9422=CARTESIAN_POINT('Ctrl Pts',(1.628621697537,101.,5.999999999856));
#9423=CARTESIAN_POINT('Ctrl Pts',(-1.689481893123,102.1196847108,6.992808061201));
#9424=CARTESIAN_POINT('Ctrl Pts',(-1.669187233917,102.1197065598,6.992808061201));
#9425=CARTESIAN_POINT('Ctrl Pts',(-1.512636201126,102.1197869626,6.992808061201));
#9426=CARTESIAN_POINT('Ctrl Pts',(-1.23556503978,102.1188276871,6.992808061201));
#9427=CARTESIAN_POINT('Ctrl Pts',(-0.8648101546223,102.1166806136,6.992808061201));
#9428=CARTESIAN_POINT('Ctrl Pts',(-0.5109811635092,102.1148120947,6.992808061201));
#9429=CARTESIAN_POINT('Ctrl Pts',(-0.1488522802808,102.1137128273,6.992808061201));
#9430=CARTESIAN_POINT('Ctrl Pts',(0.2394130054686,102.1138378158,6.992808061201));
#9431=CARTESIAN_POINT('Ctrl Pts',(0.663639050088,102.1154833678,6.992808061201));
#9432=CARTESIAN_POINT('Ctrl Pts',(1.130096203131,102.1183003163,6.992808061201));
#9433=CARTESIAN_POINT('Ctrl Pts',(1.477116016106,102.1198046106,6.992808061201));
#9434=CARTESIAN_POINT('Ctrl Pts',(1.669209716084,102.1197066226,6.992808061201));
#9435=CARTESIAN_POINT('Ctrl Pts',(1.689515664192,102.1196849348,6.992808061201));
#9436=CARTESIAN_POINT('Ctrl Pts',(-1.688715228218,101.4207068678,7.077093790264));
#9437=CARTESIAN_POINT('Ctrl Pts',(-1.668689128932,101.4207284853,7.077093790264));
#9438=CARTESIAN_POINT('Ctrl Pts',(-1.514109227167,101.4208080916,7.077093790264));
#9439=CARTESIAN_POINT('Ctrl Pts',(-1.239188923109,101.4198586149,7.077093790264));
#9440=CARTESIAN_POINT('Ctrl Pts',(-0.8689370512758,101.41771466,7.077093790264));
#9441=CARTESIAN_POINT('Ctrl Pts',(-0.5140416525734,101.4158400361,7.077093790264));
#9442=CARTESIAN_POINT('Ctrl Pts',(-0.1498433242845,101.4147339759,7.077093790264));
#9443=CARTESIAN_POINT('Ctrl Pts',(0.2409905058727,101.4148598525,7.077093790264));
#9444=CARTESIAN_POINT('Ctrl Pts',(0.667428084141,101.4165149357,7.077093790264));
#9445=CARTESIAN_POINT('Ctrl Pts',(1.134325060388,101.4193353122,7.077093790264));
#9446=CARTESIAN_POINT('Ctrl Pts',(1.479036591025,101.4208256727,7.077093790264));
#9447=CARTESIAN_POINT('Ctrl Pts',(1.668711295896,101.4207285315,7.077093790264));
#9448=CARTESIAN_POINT('Ctrl Pts',(1.688748453112,101.4207070467,7.077093790264));
#9449=CARTESIAN_POINT('Ctrl Pts',(-1.68816918717,100.9228745154,6.579261201271));
#9450=CARTESIAN_POINT('Ctrl Pts',(-1.668334364073,100.922895968,6.579261201271));
#9451=CARTESIAN_POINT('Ctrl Pts',(-1.515158359163,100.9229750071,6.579261201271));
#9452=CARTESIAN_POINT('Ctrl Pts',(-1.241769958231,100.9220325094,6.579261201271));
#9453=CARTESIAN_POINT('Ctrl Pts',(-0.8718763471198,100.9198907756,6.579261201271));
#9454=CARTESIAN_POINT('Ctrl Pts',(-0.5162214219115,100.9180118035,6.579261201271));
#9455=CARTESIAN_POINT('Ctrl Pts',(-0.1505491746523,100.9169009054,6.579261201271));
#9456=CARTESIAN_POINT('Ctrl Pts',(0.2421140475483,100.9170274144,6.579261201271));
#9457=CARTESIAN_POINT('Ctrl Pts',(0.6701267444128,100.918689286,6.579261201271));
#9458=CARTESIAN_POINT('Ctrl Pts',(1.137336975539,100.9215121041,6.579261201271));
#9459=CARTESIAN_POINT('Ctrl Pts',(1.480404480349,100.9229925405,6.579261201271));
#9460=CARTESIAN_POINT('Ctrl Pts',(1.668356306539,100.9228960023,6.579261201271));
#9461=CARTESIAN_POINT('Ctrl Pts',(1.688202023064,100.9228746621,6.579261201271));
#9462=CARTESIAN_POINT('Ctrl Pts',(-1.688261634851,101.0071602049,5.880283026469));
#9463=CARTESIAN_POINT('Ctrl Pts',(-1.668394427668,101.0071816854,5.880283026469));
#9464=CARTESIAN_POINT('Ctrl Pts',(-1.514980735485,101.0072608205,5.880283026469));
#9465=CARTESIAN_POINT('Ctrl Pts',(-1.241332975131,101.0063171412,5.880283026469));
#9466=CARTESIAN_POINT('Ctrl Pts',(-0.8713787085563,101.0041750314,5.880283026469));
#9467=CARTESIAN_POINT('Ctrl Pts',(-0.5158523752623,101.0022967954,5.880283026469));
#9468=CARTESIAN_POINT('Ctrl Pts',(-0.1504296703963,101.0011867164,5.880283026469));
#9469=CARTESIAN_POINT('Ctrl Pts',(0.2419238259119,101.0013131184,5.880283026469));
#9470=CARTESIAN_POINT('Ctrl Pts',(0.6696698467433,101.0029738406,5.880283026469));
#9471=CARTESIAN_POINT('Ctrl Pts',(1.136827042137,101.0057962454,5.880283026469));
#9472=CARTESIAN_POINT('Ctrl Pts',(1.480172889344,101.007278362,5.880283026469));
#9473=CARTESIAN_POINT('Ctrl Pts',(1.668416408143,101.0071817217,5.880283026469));
#9474=CARTESIAN_POINT('Ctrl Pts',(1.688294536604,101.007160357,5.880283026469));
#9475=CARTESIAN_POINT('Origin',(-1.628604434127,102.,6.));
#9476=CARTESIAN_POINT('Origin',(1.628621700447,102.,6.));
#9477=CARTESIAN_POINT('Origin',(-8.153768,102.,6.));
#9478=CARTESIAN_POINT('Origin',(7.,102.,6.));
#9479=CARTESIAN_POINT('Origin',(7.,102.,6.));
#9480=CARTESIAN_POINT('Origin',(-75.7512,102.,6.));
#9481=CARTESIAN_POINT('Origin',(-7.,102.,6.));
#9482=CARTESIAN_POINT('Origin',(-7.,102.,6.));
#9483=CARTESIAN_POINT('',(-8.,102.,6.));
#9484=CARTESIAN_POINT('Origin',(-7.,102.,6.));
#9485=CARTESIAN_POINT('Origin',(-7.,102.,6.));
#9486=CARTESIAN_POINT('Origin',(-7.,102.,43.78380184031));
#9487=CARTESIAN_POINT('',(-8.,102.,-6.));
#9488=CARTESIAN_POINT('',(-8.,102.,6.));
#9489=CARTESIAN_POINT('Origin',(-7.,102.,-6.));
#9490=CARTESIAN_POINT('Origin',(-7.,102.,-6.));
#9491=CARTESIAN_POINT('Origin',(-7.,102.,-6.));
#9492=CARTESIAN_POINT('Origin',(-7.,-138.3504337905,-6.));
#9493=CARTESIAN_POINT('',(-8.,116.,-6.));
#9494=CARTESIAN_POINT('',(-8.,102.,-6.));
#9495=CARTESIAN_POINT('Origin',(-7.,116.,-6.));
#9496=CARTESIAN_POINT('Origin',(-8.,117.,-7.));
#9497=CARTESIAN_POINT('',(-8.,116.,6.));
#9498=CARTESIAN_POINT('',(-8.,116.,6.));
#9499=CARTESIAN_POINT('',(-8.,116.,6.));
#9500=CARTESIAN_POINT('Origin',(-7.,116.,43.78380184031));
#9501=CARTESIAN_POINT('',(-7.,117.,6.));
#9502=CARTESIAN_POINT('Origin',(-7.,116.,6.));
#9503=CARTESIAN_POINT('',(-7.,117.,-6.));
#9504=CARTESIAN_POINT('',(-7.,117.,6.));
#9505=CARTESIAN_POINT('Origin',(-7.,116.,-6.));
#9506=CARTESIAN_POINT('Origin',(-7.,116.,-6.));
#9507=CARTESIAN_POINT('Origin',(-7.,116.,-6.));
#9508=CARTESIAN_POINT('Origin',(-75.7512,116.,-6.));
#9509=CARTESIAN_POINT('',(7.,117.,-6.));
#9510=CARTESIAN_POINT('',(-7.,117.,-6.));
#9511=CARTESIAN_POINT('Origin',(7.,116.,-6.));
#9512=CARTESIAN_POINT('Origin',(7.,116.,-6.));
#9513=CARTESIAN_POINT('Origin',(7.,116.,-6.));
#9514=CARTESIAN_POINT('Origin',(7.,116.,-6.));
#9515=CARTESIAN_POINT('Origin',(7.,269.5212,-6.));
#9516=CARTESIAN_POINT('Origin',(7.,116.,43.78380184031));
#9517=CARTESIAN_POINT('',(7.,117.,6.));
#9518=CARTESIAN_POINT('',(7.,117.,6.));
#9519=CARTESIAN_POINT('Origin',(7.,116.,6.));
#9520=CARTESIAN_POINT('Origin',(8.,117.,-7.));
#9521=CARTESIAN_POINT('',(7.,117.,6.));
#9522=CARTESIAN_POINT('',(-4.,117.,4.89858719658941E-16));
#9523=CARTESIAN_POINT('Origin',(0.,117.,0.));
#9524=CARTESIAN_POINT('Origin',(75.7512,116.,6.));
#9525=CARTESIAN_POINT('Origin',(-7.,116.,6.));
#9526=CARTESIAN_POINT('Origin',(7.,116.,6.));
#9527=CARTESIAN_POINT('Origin',(7.,116.,6.));
#9528=CARTESIAN_POINT('Origin',(-7.,116.,6.));
#9529=CARTESIAN_POINT('Origin',(-7.,116.,6.));
#9530=CARTESIAN_POINT('Origin',(-7.,269.5212,6.));
#9531=CARTESIAN_POINT('Origin',(0.,117.,0.));
#9532=CARTESIAN_POINT('',(-4.,120.,4.89858719658941E-16));
#9533=CARTESIAN_POINT('Origin',(0.,120.,0.));
#9534=CARTESIAN_POINT('',(-4.,117.,4.89858719658941E-16));
#9535=CARTESIAN_POINT('Origin',(0.,120.,-7.));
#9536=CARTESIAN_POINT('',(-1.5,120.,1.83697019872103E-16));
#9537=CARTESIAN_POINT('Origin',(0.,120.,0.));
#9538=CARTESIAN_POINT('Origin',(0.,119.875,0.));
#9539=CARTESIAN_POINT('',(-1.25,119.75,1.5308084989342E-16));
#9540=CARTESIAN_POINT('Origin',(0.,119.75,0.));
#9541=CARTESIAN_POINT('',(-1.375,119.875,1.68388934882761E-16));
#9542=CARTESIAN_POINT('Origin',(0.,109.7613704375,0.));
#9543=CARTESIAN_POINT('',(-1.25,109.7613704375,1.53080849893419E-16));
#9544=CARTESIAN_POINT('Origin',(0.,69.72097410502,0.));
#9545=CARTESIAN_POINT('',(0.,47.91425627512,6.712116818331));
#9546=CARTESIAN_POINT('',(6.71211681833062,47.91425627512,8.21997237707171E-16));
#9547=CARTESIAN_POINT('Origin',(0.,47.91425627512,0.));
#9548=CARTESIAN_POINT('',(5.187242561534,69.72097410502,6.35253999938353E-16));
#9549=CARTESIAN_POINT('Origin',(0.,47.91425627512,0.));
#9550=CARTESIAN_POINT('Origin',(0.,69.72097410502,0.));
#9551=CARTESIAN_POINT('',(7.15007114377336,41.65121763128,8.75631173989789E-16));
#9552=CARTESIAN_POINT('',(0.0106247171632265,41.65121763128,7.15006324981918));
#9553=CARTESIAN_POINT('Origin',(0.,41.65121763128,0.));
#9554=CARTESIAN_POINT('Origin',(0.,41.65121763128,0.));
#9555=CARTESIAN_POINT('',(7.11077262920686,42.2132125724799,8.70818493982279E-16));
#9556=CARTESIAN_POINT('',(5.187242561534,69.72097410502,6.35253999938353E-16));
#9557=CARTESIAN_POINT('',(0.,42.21321257248,7.110772629208));
#9558=CARTESIAN_POINT('Origin',(0.,42.21321257248,0.));
#9559=CARTESIAN_POINT('Origin',(0.,42.21321257248,0.));
#9560=CARTESIAN_POINT('Origin',(0.,45.,0.));
#9561=CARTESIAN_POINT('Origin',(7.34788079488412E-16,45.,6.));
#9562=CARTESIAN_POINT('Origin',(0.,42.,0.));
#9563=CARTESIAN_POINT('',(0.011887692143076,39.1932353328207,8.00000000000279));
#9564=CARTESIAN_POINT('Origin',(0.0180364167624925,42.,12.1378779943689));
#9565=CARTESIAN_POINT('',(9.1284394897767,37.,8.));
#9566=CARTESIAN_POINT('Ctrl Pts',(9.12843948977668,37.,8.));
#9567=CARTESIAN_POINT('Ctrl Pts',(8.57403140594617,37.,8.));
#9568=CARTESIAN_POINT('Ctrl Pts',(7.96896895550773,37.0558564477204,8.));
#9569=CARTESIAN_POINT('Ctrl Pts',(6.77413711943837,37.2666014130387,8.));
#9570=CARTESIAN_POINT('Ctrl Pts',(6.18411009233275,37.4200265971388,8.));
#9571=CARTESIAN_POINT('Ctrl Pts',(4.75709729947724,37.8565700407443,8.));
#9572=CARTESIAN_POINT('Ctrl Pts',(3.80441040251253,38.2365947939282,8.));
#9573=CARTESIAN_POINT('Ctrl Pts',(1.90336768275116,38.9163280810235,8.));
#9574=CARTESIAN_POINT('Ctrl Pts',(0.946007958016012,39.1911889725053,8.));
#9575=CARTESIAN_POINT('Ctrl Pts',(0.0118876940187937,39.1932353328207,8.));
#9576=CARTESIAN_POINT('',(11.0000000430061,36.9999999999999,5.13112121888498));
#9577=CARTESIAN_POINT('Origin',(0.,37.,0.));
#9578=CARTESIAN_POINT('',(11.1896485656096,37.0907398175677,-0.000169479335991176));
#9579=CARTESIAN_POINT('Ctrl Pts',(11.0000000164978,36.9999999999997,5.13112121714035));
#9580=CARTESIAN_POINT('Ctrl Pts',(11.0111825439989,36.9999999953411,4.96121154043948));
#9581=CARTESIAN_POINT('Ctrl Pts',(11.0218701867737,37.0011359668517,4.79400389659548));
#9582=CARTESIAN_POINT('Ctrl Pts',(11.0320046124329,37.0030129927172,4.63027386211126));
#9583=CARTESIAN_POINT('Ctrl Pts',(11.0387890381477,37.0042695555436,4.52066584942374));
#9584=CARTESIAN_POINT('Ctrl Pts',(11.0453260204498,37.0058588915485,4.41261648872546));
#9585=CARTESIAN_POINT('Ctrl Pts',(11.0516043222841,37.0076742438597,4.30635962787506));
#9586=CARTESIAN_POINT('Ctrl Pts',(11.0588074658838,37.0097570114179,4.18445032065147));
#9587=CARTESIAN_POINT('Ctrl Pts',(11.065661238494,37.0121352203763,4.06489359579171));
#9588=CARTESIAN_POINT('Ctrl Pts',(11.072247928066,37.0147222240793,3.94622081445611));
#9589=CARTESIAN_POINT('Ctrl Pts',(11.0795239743893,37.0175799811627,3.81512785115984));
#9590=CARTESIAN_POINT('Ctrl Pts',(11.0864749761023,37.0206940009696,3.68511373779337));
#9591=CARTESIAN_POINT('Ctrl Pts',(11.0931851556689,37.0239939869192,3.55417020202618));
#9592=CARTESIAN_POINT('Ctrl Pts',(11.0936038808397,37.0241999109435,3.54599913091845));
#9593=CARTESIAN_POINT('Ctrl Pts',(11.0940216577092,37.024406568043,3.53782443170898));
#9594=CARTESIAN_POINT('Ctrl Pts',(11.0944385023882,37.0246139441538,3.52964561286928));
#9595=CARTESIAN_POINT('Ctrl Pts',(11.1035557560452,37.0291496878003,3.35075796061484));
#9596=CARTESIAN_POINT('Ctrl Pts',(11.1122444065986,37.0340295031561,3.16991671730982));
#9597=CARTESIAN_POINT('Ctrl Pts',(11.1204316981979,37.0390274579943,2.98613137636941));
#9598=CARTESIAN_POINT('Ctrl Pts',(11.1240477545458,37.0412348896096,2.90495946002643));
#9599=CARTESIAN_POINT('Ctrl Pts',(11.1275655528008,37.0434650373592,2.82321306518882));
#9600=CARTESIAN_POINT('Ctrl Pts',(11.1309764107165,37.0456961209886,2.74080610561445));
#9601=CARTESIAN_POINT('Ctrl Pts',(11.1376689356853,37.0500737829335,2.57911346165467));
#9602=CARTESIAN_POINT('Ctrl Pts',(11.1439502033684,37.05445742758,2.41487893318168));
#9603=CARTESIAN_POINT('Ctrl Pts',(11.1497597449324,37.0586941757249,2.24739586736983));
#9604=CARTESIAN_POINT('Ctrl Pts',(11.1536148395963,37.0615055963827,2.1362574812872));
#9605=CARTESIAN_POINT('Ctrl Pts',(11.1572616759657,37.0642517494188,2.02368854786336));
#9606=CARTESIAN_POINT('Ctrl Pts',(11.1606749001187,37.0668775563969,1.90948220592755));
#9607=CARTESIAN_POINT('Ctrl Pts',(11.1649533384812,37.0701689761234,1.76632583157622));
#9608=CARTESIAN_POINT('Ctrl Pts',(11.1688593820582,37.0732744443208,1.62059725365725));
#9609=CARTESIAN_POINT('Ctrl Pts',(11.1723451311472,37.0761105840506,1.47105010106573));
#9610=CARTESIAN_POINT('Ctrl Pts',(11.1755030580699,37.0786799950381,1.33556732037411));
#9611=CARTESIAN_POINT('Ctrl Pts',(11.1783159006795,37.0810286574292,1.19695011526774));
#9612=CARTESIAN_POINT('Ctrl Pts',(11.1807164562182,37.0830600739771,1.05427204426782));
#9613=CARTESIAN_POINT('Ctrl Pts',(11.1809656561954,37.083270953896,1.03946073435624));
#9614=CARTESIAN_POINT('Ctrl Pts',(11.1812103833398,37.0834783790926,1.02460566578708));
#9615=CARTESIAN_POINT('Ctrl Pts',(11.1814505411601,37.0836822154566,1.00970580448101));
#9616=CARTESIAN_POINT('Ctrl Pts',(11.1844070041638,37.086191543149,0.826281052145604));
#9617=CARTESIAN_POINT('Ctrl Pts',(11.1866861367669,37.0881564592366,0.636073731167722));
#9618=CARTESIAN_POINT('Ctrl Pts',(11.1880832646347,37.0893710087782,0.439358371355146));
#9619=CARTESIAN_POINT('Ctrl Pts',(11.1890996419792,37.0902545647264,0.296252618727001));
#9620=CARTESIAN_POINT('Ctrl Pts',(11.1896489896218,37.0907404613239,0.149703434419743));
#9621=CARTESIAN_POINT('Ctrl Pts',(11.1896485656097,37.0907398175686,-0.000169479335990849));
#9622=CARTESIAN_POINT('',(11.00000001131,36.9999999999996,-5.1311213989913));
#9623=CARTESIAN_POINT('Ctrl Pts',(11.1896485656095,37.0907398175672,-0.000169481921701897));
#9624=CARTESIAN_POINT('Ctrl Pts',(11.1896479776106,37.0907393489086,-0.215681937420152));
#9625=CARTESIAN_POINT('Ctrl Pts',(11.1885084096789,37.0897437526926,-0.429458199024161));
#9626=CARTESIAN_POINT('Ctrl Pts',(11.1863420983071,37.0878649344339,-0.640356926161641));
#9627=CARTESIAN_POINT('Ctrl Pts',(11.1848579333,37.0865777342879,-0.784846086366657));
#9628=CARTESIAN_POINT('Ctrl Pts',(11.1828937972378,37.0848807618758,-0.927983658842167));
#9629=CARTESIAN_POINT('Ctrl Pts',(11.1804313296578,37.0828103697687,-1.07149129532294));
#9630=CARTESIAN_POINT('Ctrl Pts',(11.1792995395267,37.0818587838987,-1.1374497379955));
#9631=CARTESIAN_POINT('Ctrl Pts',(11.1780624885594,37.0808275508911,-1.20348625455482));
#9632=CARTESIAN_POINT('Ctrl Pts',(11.1767184554982,37.079716688106,-1.26976720008837));
#9633=CARTESIAN_POINT('Ctrl Pts',(11.1737179373486,37.0772367164114,-1.41773765244469));
#9634=CARTESIAN_POINT('Ctrl Pts',(11.170180947628,37.0743547381601,-1.56692968835248));
#9635=CARTESIAN_POINT('Ctrl Pts',(11.1661975793124,37.0711980429517,-1.71481587196975));
#9636=CARTESIAN_POINT('Ctrl Pts',(11.1645145444965,37.0698642903287,-1.77730007531386));
#9637=CARTESIAN_POINT('Ctrl Pts',(11.162751830014,37.068482172809,-1.83955138112467));
#9638=CARTESIAN_POINT('Ctrl Pts',(11.1609162604204,37.0670636502293,-1.90138036125891));
#9639=CARTESIAN_POINT('Ctrl Pts',(11.1556956020255,37.0630291413554,-2.07723203439244));
#9640=CARTESIAN_POINT('Ctrl Pts',(11.1498881311807,37.05870533442,-2.24966268054424));
#9641=CARTESIAN_POINT('Ctrl Pts',(11.1435805979118,37.0542623608385,-2.41970231738112));
#9642=CARTESIAN_POINT('Ctrl Pts',(11.1424215894495,37.0534459649894,-2.45094707973465));
#9643=CARTESIAN_POINT('Ctrl Pts',(11.1412457008067,37.0526254051766,-2.48211109005339));
#9644=CARTESIAN_POINT('Ctrl Pts',(11.1400534753533,37.0518015675164,-2.51320070664233));
#9645=CARTESIAN_POINT('Ctrl Pts',(11.1340795973032,37.0476735683188,-2.66898129125717));
#9646=CARTESIAN_POINT('Ctrl Pts',(11.1276955664116,37.0434656559455,-2.82289198400398));
#9647=CARTESIAN_POINT('Ctrl Pts',(11.1207794793186,37.0392364138983,-2.97845296202742));
#9648=CARTESIAN_POINT('Ctrl Pts',(11.118803649819,37.0380281785066,-3.02289456104516));
#9649=CARTESIAN_POINT('Ctrl Pts',(11.1167844246291,37.0368181061012,-3.06747053813211));
#9650=CARTESIAN_POINT('Ctrl Pts',(11.1147190384397,37.0356076179028,-3.11226217733893));
#9651=CARTESIAN_POINT('Ctrl Pts',(11.1083673846949,37.0318850201926,-3.25000928941724));
#9652=CARTESIAN_POINT('Ctrl Pts',(11.101578293801,37.0281556654332,-3.3897989420054));
#9653=CARTESIAN_POINT('Ctrl Pts',(11.0942772760587,37.0245331428097,-3.53281226756565));
#9654=CARTESIAN_POINT('Ctrl Pts',(11.0908940504137,37.0228544985615,-3.59908335026864));
#9655=CARTESIAN_POINT('Ctrl Pts',(11.0874009596442,37.0211993154306,-3.66604635730229));
#9656=CARTESIAN_POINT('Ctrl Pts',(11.0837909632952,37.0195825443791,-3.73381714784607));
#9657=CARTESIAN_POINT('Ctrl Pts',(11.0771004661201,37.0165861418603,-3.85941846121413));
#9658=CARTESIAN_POINT('Ctrl Pts',(11.0700080901534,37.0137189253489,-3.98779522803996));
#9659=CARTESIAN_POINT('Ctrl Pts',(11.0624744656947,37.0111220264858,-4.11941195521222));
#9660=CARTESIAN_POINT('Ctrl Pts',(11.0571710426893,37.0092938953851,-4.21206578772226));
#9661=CARTESIAN_POINT('Ctrl Pts',(11.0516490173313,37.0076004516683,-4.30632503899295));
#9662=CARTESIAN_POINT('Ctrl Pts',(11.0458959603966,37.0061063072661,-4.40234852950457));
#9663=CARTESIAN_POINT('Ctrl Pts',(11.0383442029163,37.0041450167219,-4.52839388608507));
#9664=CARTESIAN_POINT('Ctrl Pts',(11.0303942662333,37.0025253678984,-4.65747976771746));
#9665=CARTESIAN_POINT('Ctrl Pts',(11.0220365153567,37.0014432233025,-4.78968265020428));
#9666=CARTESIAN_POINT('Ctrl Pts',(11.0149826233968,37.0005298997089,-4.90126109560603));
#9667=CARTESIAN_POINT('Ctrl Pts',(11.0076382775635,36.9999999853001,-5.01505974973993));
#9668=CARTESIAN_POINT('Ctrl Pts',(11.000000004389,36.9999999999982,-5.13112139853582));
#9669=CARTESIAN_POINT('',(9.12843948977674,36.9999999999999,-8.00000000000001));
#9670=CARTESIAN_POINT('Origin',(0.,37.,0.));
#9671=CARTESIAN_POINT('',(-9.12843948977662,37.,-8.00000000000001));
#9672=CARTESIAN_POINT('Ctrl Pts',(-9.12843948977668,37.,-8.));
#9673=CARTESIAN_POINT('Ctrl Pts',(-8.57403140594617,37.,-8.));
#9674=CARTESIAN_POINT('Ctrl Pts',(-7.96896895550773,37.0558564477204,-8.));
#9675=CARTESIAN_POINT('Ctrl Pts',(-6.77413711943837,37.2666014130387,-8.));
#9676=CARTESIAN_POINT('Ctrl Pts',(-6.18411009233275,37.4200265971388,-8.));
#9677=CARTESIAN_POINT('Ctrl Pts',(-4.75709729947724,37.8565700407443,-8.));
#9678=CARTESIAN_POINT('Ctrl Pts',(-3.80441040251253,38.2365947939282,-8.));
#9679=CARTESIAN_POINT('Ctrl Pts',(-1.89934365236072,38.9177669058201,-8.));
#9680=CARTESIAN_POINT('Ctrl Pts',(-0.937884008599215,39.1932483539498,-8.));
#9681=CARTESIAN_POINT('Ctrl Pts',(0.,39.1932483539498,-8.));
#9682=CARTESIAN_POINT('Ctrl Pts',(0.937884008599215,39.1932483539498,-8.));
#9683=CARTESIAN_POINT('Ctrl Pts',(1.89934365236072,38.9177669058201,-8.));
#9684=CARTESIAN_POINT('Ctrl Pts',(3.80441040251253,38.2365947939282,-8.));
#9685=CARTESIAN_POINT('Ctrl Pts',(4.75709729947724,37.8565700407443,-8.));
#9686=CARTESIAN_POINT('Ctrl Pts',(6.18411009233275,37.4200265971388,-8.));
#9687=CARTESIAN_POINT('Ctrl Pts',(6.77413711943837,37.2666014130387,-8.));
#9688=CARTESIAN_POINT('Ctrl Pts',(7.96896895550773,37.0558564477204,-8.));
#9689=CARTESIAN_POINT('Ctrl Pts',(8.57403140594617,37.,-8.));
#9690=CARTESIAN_POINT('Ctrl Pts',(9.12843948977668,37.,-8.));
#9691=CARTESIAN_POINT('',(-11.0000003498417,36.9999999999996,-5.13111944275097));
#9692=CARTESIAN_POINT('Origin',(0.,37.,0.));
#9693=CARTESIAN_POINT('',(-11.0000000676958,36.9999999999997,5.1311211208313));
#9694=CARTESIAN_POINT('Ctrl Pts',(-11.00000002783,36.9999999999987,5.131121044419));
#9695=CARTESIAN_POINT('Ctrl Pts',(-11.0140712521959,36.9999998982868,4.91732288718392));
#9696=CARTESIAN_POINT('Ctrl Pts',(-11.0276242001948,37.0017973389252,4.70395369933127));
#9697=CARTESIAN_POINT('Ctrl Pts',(-11.0405748924402,37.0047974379781,4.49058332358683));
#9698=CARTESIAN_POINT('Ctrl Pts',(-11.0469128280474,37.0062656556033,4.38616205587838));
#9699=CARTESIAN_POINT('Ctrl Pts',(-11.0531064872421,37.0080228023865,4.28174026543605));
#9700=CARTESIAN_POINT('Ctrl Pts',(-11.0591455982534,37.0100032565513,4.17726625883438));
#9701=CARTESIAN_POINT('Ctrl Pts',(-11.0775247948997,37.0160304940826,3.85931411187551));
#9702=CARTESIAN_POINT('Ctrl Pts',(-11.0944748101117,37.0241218487547,3.54088391180374));
#9703=CARTESIAN_POINT('Ctrl Pts',(-11.1095943066205,37.0326593422877,3.22184910859468));
#9704=CARTESIAN_POINT('Ctrl Pts',(-11.1187140108614,37.0378089460416,3.02941525035502));
#9705=CARTESIAN_POINT('Ctrl Pts',(-11.1271734995192,37.0431206795202,2.8367637002585));
#9706=CARTESIAN_POINT('Ctrl Pts',(-11.134861631142,37.0482731329454,2.64520456823093));
#9707=CARTESIAN_POINT('Ctrl Pts',(-11.1399196013838,37.051662897504,2.51917909977126));
#9708=CARTESIAN_POINT('Ctrl Pts',(-11.1446444463466,37.0549837079099,2.39362690391072));
#9709=CARTESIAN_POINT('Ctrl Pts',(-11.1490146449952,37.0581507000346,2.26892480975772));
#9710=CARTESIAN_POINT('Ctrl Pts',(-11.1549415540522,37.0624458078356,2.0998025270654));
#9711=CARTESIAN_POINT('Ctrl Pts',(-11.1602029823346,37.066463069481,1.93223807087765));
#9712=CARTESIAN_POINT('Ctrl Pts',(-11.1648420582513,37.0701137654189,1.76477567623669));
#9713=CARTESIAN_POINT('Ctrl Pts',(-11.1688229474782,37.0732465048677,1.62107265117187));
#9714=CARTESIAN_POINT('Ctrl Pts',(-11.1723450969853,37.0761098710538,1.47744412273924));
#9715=CARTESIAN_POINT('Ctrl Pts',(-11.1754100328185,37.0786343854209,1.33295994640686));
#9716=CARTESIAN_POINT('Ctrl Pts',(-11.1787283416866,37.081367597099,1.17653150883889));
#9717=CARTESIAN_POINT('Ctrl Pts',(-11.1815094557598,37.0837049268536,1.01910414823258));
#9718=CARTESIAN_POINT('Ctrl Pts',(-11.1837157609282,37.0855863364246,0.859408825005803));
#9719=CARTESIAN_POINT('Ctrl Pts',(-11.1857777329768,37.0873446670504,0.710160526304185));
#9720=CARTESIAN_POINT('Ctrl Pts',(-11.1873375402417,37.0887050572166,0.558930819716984));
#9721=CARTESIAN_POINT('Ctrl Pts',(-11.1883298687427,37.0895851698554,0.40468523977506));
#9722=CARTESIAN_POINT('Ctrl Pts',(-11.1883993293682,37.0896467756385,0.393888417495881));
#9723=CARTESIAN_POINT('Ctrl Pts',(-11.188465994842,37.0897060127454,0.383076820735572));
#9724=CARTESIAN_POINT('Ctrl Pts',(-11.1885298360109,37.089762845708,0.372250095909413));
#9725=CARTESIAN_POINT('Ctrl Pts',(-11.1893515624725,37.0904943666063,0.232894779729622));
#9726=CARTESIAN_POINT('Ctrl Pts',(-11.1897251319801,37.0908203025814,0.091033038055436));
#9727=CARTESIAN_POINT('Ctrl Pts',(-11.1896061673193,37.0907133376148,-0.051869431910791));
#9728=CARTESIAN_POINT('Ctrl Pts',(-11.1894871572608,37.0906063318296,-0.194826434508157));
#9729=CARTESIAN_POINT('Ctrl Pts',(-11.1888751656669,37.0900661047587,-0.338824405220953));
#9730=CARTESIAN_POINT('Ctrl Pts',(-11.187764938011,37.0890997865693,-0.482392709589935));
#9731=CARTESIAN_POINT('Ctrl Pts',(-11.1873489450846,37.0887377153046,-0.53618654075308));
#9732=CARTESIAN_POINT('Ctrl Pts',(-11.1868634011007,37.0883161682624,-0.589920059916406));
#9733=CARTESIAN_POINT('Ctrl Pts',(-11.1863094553398,37.0878367426741,-0.64351603627636));
#9734=CARTESIAN_POINT('Ctrl Pts',(-11.184708991504,37.0864515830243,-0.798365893382707));
#9735=CARTESIAN_POINT('Ctrl Pts',(-11.1825307099028,37.0845819711465,-0.952073832901876));
#9736=CARTESIAN_POINT('Ctrl Pts',(-11.1798663337782,37.0823448383766,-1.10299844583809));
#9737=CARTESIAN_POINT('Ctrl Pts',(-11.1770641026185,37.079991956177,-1.26173191039888));
#9738=CARTESIAN_POINT('Ctrl Pts',(-11.1737243966345,37.0772335467755,-1.41738578506559));
#9739=CARTESIAN_POINT('Ctrl Pts',(-11.1700003378975,37.0742288059789,-1.56807286505966));
#9740=CARTESIAN_POINT('Ctrl Pts',(-11.1694993295277,37.0738245695277,-1.58834523282626));
#9741=CARTESIAN_POINT('Ctrl Pts',(-11.1689914265003,37.0734158935885,-1.60852774786708));
#9742=CARTESIAN_POINT('Ctrl Pts',(-11.1684770570016,37.0730031797098,-1.6286158554092));
#9743=CARTESIAN_POINT('Ctrl Pts',(-11.1647599161538,37.0700206630152,-1.77378450421377));
#9744=CARTESIAN_POINT('Ctrl Pts',(-11.160686642056,37.0668348340176,-1.91401538308741));
#9745=CARTESIAN_POINT('Ctrl Pts',(-11.1563544893698,37.0635682346049,-2.04984526937032));
#9746=CARTESIAN_POINT('Ctrl Pts',(-11.1516936488259,37.0600537926897,-2.19598080219131));
#9747=CARTESIAN_POINT('Ctrl Pts',(-11.1467331069504,37.0564454021741,-2.33702237230987));
#9748=CARTESIAN_POINT('Ctrl Pts',(-11.1415612051114,37.0528467225342,-2.47364127210357));
#9749=CARTESIAN_POINT('Ctrl Pts',(-11.1412292039677,37.052615711623,-2.4824112821301));
#9750=CARTESIAN_POINT('Ctrl Pts',(-11.1408963216095,37.0523847266039,-2.49116306766433));
#9751=CARTESIAN_POINT('Ctrl Pts',(-11.1405625772943,37.0521537893321,-2.49989680636301));
#9752=CARTESIAN_POINT('Ctrl Pts',(-11.134890548819,37.0482289800629,-2.64832784276284));
#9753=CARTESIAN_POINT('Ctrl Pts',(-11.1289763642823,37.044321766251,-2.79154494313647));
#9754=CARTESIAN_POINT('Ctrl Pts',(-11.1229071577116,37.0405521348536,-2.9300690866496));
#9755=CARTESIAN_POINT('Ctrl Pts',(-11.1178853359213,37.0374330422883,-3.04468762109334));
#9756=CARTESIAN_POINT('Ctrl Pts',(-11.1127566977551,37.0344068277067,-3.15609321605914));
#9757=CARTESIAN_POINT('Ctrl Pts',(-11.1075567552947,37.0315187150892,-3.26458007893159));
#9758=CARTESIAN_POINT('Ctrl Pts',(-11.1004464312207,37.0275695527995,-3.41292340362817));
#9759=CARTESIAN_POINT('Ctrl Pts',(-11.0932054709357,37.0238800107333,-3.55580866728893));
#9760=CARTESIAN_POINT('Ctrl Pts',(-11.0859024624725,37.0205377067675,-3.69402073450888));
#9761=CARTESIAN_POINT('Ctrl Pts',(-11.0814098321309,37.0184816039595,-3.7790453828982));
#9762=CARTESIAN_POINT('Ctrl Pts',(-11.0768930183602,37.0165558606314,-3.86230134249087));
#9763=CARTESIAN_POINT('Ctrl Pts',(-11.0723622744047,37.0147735012423,-3.94396971338329));
#9764=CARTESIAN_POINT('Ctrl Pts',(-11.0638397053627,37.0114207889504,-4.0975922390254));
#9765=CARTESIAN_POINT('Ctrl Pts',(-11.055271239492,37.008575969418,-4.24559707805008));
#9766=CARTESIAN_POINT('Ctrl Pts',(-11.0466513754209,37.0063032181303,-4.38975182817902));
#9767=CARTESIAN_POINT('Ctrl Pts',(-11.0432397280449,37.0054036881721,-4.44680669249741));
#9768=CARTESIAN_POINT('Ctrl Pts',(-11.0398195142528,37.004593589514,-4.50325814803838));
#9769=CARTESIAN_POINT('Ctrl Pts',(-11.0363885793265,37.0038767568708,-4.5592146232255));
#9770=CARTESIAN_POINT('Ctrl Pts',(-11.0281541333304,37.0021563162868,-4.69351346099501));
#9771=CARTESIAN_POINT('Ctrl Pts',(-11.0198635189573,37.0009770903936,-4.82496577179628));
#9772=CARTESIAN_POINT('Ctrl Pts',(-11.0116031991166,37.0004045381099,-4.95304618956424));
#9773=CARTESIAN_POINT('Ctrl Pts',(-11.0077259733317,37.0001357937368,-5.01316452733983));
#9774=CARTESIAN_POINT('Ctrl Pts',(-11.0038553876797,36.9999999968381,-5.0725401265193));
#9775=CARTESIAN_POINT('Ctrl Pts',(-11.0000001341984,36.9999999999985,-5.13111942855892));
#9776=CARTESIAN_POINT('',(-9.12843948977677,37.,8.00000000000001));
#9777=CARTESIAN_POINT('Origin',(0.,37.,0.));
#9778=CARTESIAN_POINT('Ctrl Pts',(0.0118876940187937,39.1932353328207,8.));
#9779=CARTESIAN_POINT('Ctrl Pts',(0.00792470899211094,39.1932440144601,
8.));
#9780=CARTESIAN_POINT('Ctrl Pts',(0.00396214332439191,39.1932483539498,
8.));
#9781=CARTESIAN_POINT('Ctrl Pts',(0.,39.1932483539498,8.));
#9782=CARTESIAN_POINT('Ctrl Pts',(-0.937884008599215,39.1932483539498,8.));
#9783=CARTESIAN_POINT('Ctrl Pts',(-1.89934365236072,38.9177669058201,8.));
#9784=CARTESIAN_POINT('Ctrl Pts',(-3.80441040251253,38.2365947939282,8.));
#9785=CARTESIAN_POINT('Ctrl Pts',(-4.75709729947724,37.8565700407443,8.));
#9786=CARTESIAN_POINT('Ctrl Pts',(-6.18411009233275,37.4200265971388,8.));
#9787=CARTESIAN_POINT('Ctrl Pts',(-6.77413711943837,37.2666014130387,8.));
#9788=CARTESIAN_POINT('Ctrl Pts',(-7.96896895550773,37.0558564477204,8.));
#9789=CARTESIAN_POINT('Ctrl Pts',(-8.57403140594617,37.,8.));
#9790=CARTESIAN_POINT('Ctrl Pts',(-9.12843948977668,37.,8.));
#9791=CARTESIAN_POINT('Ctrl Pts',(-11.99357518999,35.88698149802,5.234127330856));
#9792=CARTESIAN_POINT('Ctrl Pts',(-11.99332528583,35.88468341677,5.199787902682));
#9793=CARTESIAN_POINT('Ctrl Pts',(-11.9906318297,35.86116870728,4.838104020626));
#9794=CARTESIAN_POINT('Ctrl Pts',(-11.98427746894,35.82995506373,4.152393802744));
#9795=CARTESIAN_POINT('Ctrl Pts',(-11.97368392242,35.80923437147,3.185041719748));
#9796=CARTESIAN_POINT('Ctrl Pts',(-11.96358545097,35.80256970675,2.237007562812));
#9797=CARTESIAN_POINT('Ctrl Pts',(-11.95575094264,35.80219571054,1.29827724728));
#9798=CARTESIAN_POINT('Ctrl Pts',(-11.95157858187,35.80318886163,0.346223922685));
#9799=CARTESIAN_POINT('Ctrl Pts',(-11.9522728448,35.80297211912,-0.619776846157));
#9800=CARTESIAN_POINT('Ctrl Pts',(-11.95764819515,35.80198588038,-1.560160325752));
#9801=CARTESIAN_POINT('Ctrl Pts',(-11.96556360283,35.80346825475,-2.425528994248));
#9802=CARTESIAN_POINT('Ctrl Pts',(-11.97385262721,35.81036052627,-3.197996220919));
#9803=CARTESIAN_POINT('Ctrl Pts',(-11.98141321701,35.82435952006,-3.892356813202));
#9804=CARTESIAN_POINT('Ctrl Pts',(-11.98781352018,35.84649412881,-4.527903781733));
#9805=CARTESIAN_POINT('Ctrl Pts',(-11.9916054427,35.86966712868,-4.968832637213));
#9806=CARTESIAN_POINT('Ctrl Pts',(-11.99332547808,35.88468592982,-5.199824834647));
#9807=CARTESIAN_POINT('Ctrl Pts',(-11.99357531375,35.88698559565,-5.234182558824));
#9808=CARTESIAN_POINT('Ctrl Pts',(-12.07325730637,36.58649630964,5.231935522022));
#9809=CARTESIAN_POINT('Ctrl Pts',(-12.07454985414,36.58402482358,5.198345177035));
#9810=CARTESIAN_POINT('Ctrl Pts',(-12.08802346863,36.55862535039,4.844356710033));
#9811=CARTESIAN_POINT('Ctrl Pts',(-12.11067089349,36.52274336209,4.169388296033));
#9812=CARTESIAN_POINT('Ctrl Pts',(-12.13520968347,36.49435585584,3.208216487448));
#9813=CARTESIAN_POINT('Ctrl Pts',(-12.15233416592,36.48062816741,2.258775260772));
#9814=CARTESIAN_POINT('Ctrl Pts',(-12.16302208196,36.4749403482,1.313089996961));
#9815=CARTESIAN_POINT('Ctrl Pts',(-12.16800326631,36.47316053362,0.3504770567543));
#9816=CARTESIAN_POINT('Ctrl Pts',(-12.1672071462,36.47340225696,-0.6273013998855));
#9817=CARTESIAN_POINT('Ctrl Pts',(-12.16060767632,36.47600423761,-1.577345655872));
#9818=CARTESIAN_POINT('Ctrl Pts',(-12.1491868573,36.48289948249,-2.447846195142));
#9819=CARTESIAN_POINT('Ctrl Pts',(-12.13442993541,36.49562105325,-3.220605537441));
#9820=CARTESIAN_POINT('Ctrl Pts',(-12.117320878,36.51507009099,-3.911064023649));
#9821=CARTESIAN_POINT('Ctrl Pts',(-12.09839358012,36.54188398296,-4.539180913286));
#9822=CARTESIAN_POINT('Ctrl Pts',(-12.08315373025,36.56780508192,-4.972303617105));
#9823=CARTESIAN_POINT('Ctrl Pts',(-12.07454836184,36.58402752374,-5.198381379176));
#9824=CARTESIAN_POINT('Ctrl Pts',(-12.07325486239,36.58650065764,-5.231989739265));
#9825=CARTESIAN_POINT('Ctrl Pts',(-11.57215740323,37.08103820478,5.230385959406));
#9826=CARTESIAN_POINT('Ctrl Pts',(-11.57454062195,37.07967329503,5.197321349729));
#9827=CARTESIAN_POINT('Ctrl Pts',(-11.5994870504,37.06582965207,4.84877474796));
#9828=CARTESIAN_POINT('Ctrl Pts',(-11.6435586348,37.04985783468,4.182159616124));
#9829=CARTESIAN_POINT('Ctrl Pts',(-11.69565427244,37.04432452161,3.226793445503));
#9830=CARTESIAN_POINT('Ctrl Pts',(-11.73517840125,37.04764655185,2.277022744067));
#9831=CARTESIAN_POINT('Ctrl Pts',(-11.76164063188,37.05329035986,1.325879474367));
#9832=CARTESIAN_POINT('Ctrl Pts',(-11.77458379446,37.05704081854,0.3542057124591));
#9833=CARTESIAN_POINT('Ctrl Pts',(-11.77248304032,37.05638513415,-0.6338817685511));
#9834=CARTESIAN_POINT('Ctrl Pts',(-11.75551354838,37.05173459499,-1.592080100557));
#9835=CARTESIAN_POINT('Ctrl Pts',(-11.72777119266,37.04673198537,-2.466389122714));
#9836=CARTESIAN_POINT('Ctrl Pts',(-11.69419554211,37.0449333804,-3.238709200815));
#9837=CARTESIAN_POINT('Ctrl Pts',(-11.65766877891,37.0483717235,-3.92545012791));
#9838=CARTESIAN_POINT('Ctrl Pts',(-11.61956020182,37.05817876104,-4.547464782103));
#9839=CARTESIAN_POINT('Ctrl Pts',(-11.59047057424,37.07083271012,-4.974754447084));
#9840=CARTESIAN_POINT('Ctrl Pts',(-11.57453798318,37.07967479041,-5.197357036162));
#9841=CARTESIAN_POINT('Ctrl Pts',(-11.57215330547,37.08104070378,-5.230439469083));
#9842=CARTESIAN_POINT('Ctrl Pts',(-10.87374875436,36.99215251132,5.230664466127));
#9843=CARTESIAN_POINT('Ctrl Pts',(-10.87593621278,36.99232733695,5.197499918042));
#9844=CARTESIAN_POINT('Ctrl Pts',(-10.89888147716,36.99463686747,4.847977172931));
#9845=CARTESIAN_POINT('Ctrl Pts',(-10.94040447592,37.00791721721,4.180934342797));
#9846=CARTESIAN_POINT('Ctrl Pts',(-10.99139323323,37.03826963338,3.226556333087));
#9847=CARTESIAN_POINT('Ctrl Pts',(-11.03135207768,37.06970660384,2.277785886756));
#9848=CARTESIAN_POINT('Ctrl Pts',(-11.05876901198,37.09465581291,1.326858364153));
#9849=CARTESIAN_POINT('Ctrl Pts',(-11.07238957763,37.10800766965,0.3545564871127));
#9850=CARTESIAN_POINT('Ctrl Pts',(-11.07016832676,37.10578545697,-0.634482238718));
#9851=CARTESIAN_POINT('Ctrl Pts',(-11.05236940635,37.08859174469,-1.593087932742));
#9852=CARTESIAN_POINT('Ctrl Pts',(-11.02381047398,37.06348554479,-2.466967558413));
#9853=CARTESIAN_POINT('Ctrl Pts',(-10.99004459132,37.03792904407,-3.23845314518));
#9854=CARTESIAN_POINT('Ctrl Pts',(-10.9542117178,37.01614834803,-3.924505970997));
#9855=CARTESIAN_POINT('Ctrl Pts',(-10.91774690885,37.00027711191,-4.546416048914));
#9856=CARTESIAN_POINT('Ctrl Pts',(-10.89058822231,36.99380152261,-4.974309597361));
#9857=CARTESIAN_POINT('Ctrl Pts',(-10.87593384298,36.99232715763,-5.197535697532));
#9858=CARTESIAN_POINT('Ctrl Pts',(-10.87374518234,36.9921524769,-5.23071811287));
#9859=CARTESIAN_POINT('',(-12.,36.0000000009788,5.13112119227213));
#9860=CARTESIAN_POINT('',(-12.,36.0000000049393,-5.131119091281));
#9861=CARTESIAN_POINT('Ctrl Pts',(-12.,36.0000000009797,5.13112119227213));
#9862=CARTESIAN_POINT('Ctrl Pts',(-11.99999999395,35.9999998123161,4.8038301627559));
#9863=CARTESIAN_POINT('Ctrl Pts',(-12.00000000281,36.0095311616598,4.1528235072652));
#9864=CARTESIAN_POINT('Ctrl Pts',(-11.99999999925,36.03866469074,3.18892578408));
#9865=CARTESIAN_POINT('Ctrl Pts',(-12.0000000002,36.07095734545,2.231869777753));
#9866=CARTESIAN_POINT('Ctrl Pts',(-11.99999999995,36.0961909677,1.315189036053));
#9867=CARTESIAN_POINT('Ctrl Pts',(-12.00000000001,36.11044635878,0.3796003502206));
#9868=CARTESIAN_POINT('Ctrl Pts',(-12.,36.10831608628,-0.6377249666603));
#9869=CARTESIAN_POINT('Ctrl Pts',(-11.99999999999,36.08871384336,-1.625489635872));
#9870=CARTESIAN_POINT('Ctrl Pts',(-12.00000000003,36.06245143419,-2.484605093247));
#9871=CARTESIAN_POINT('Ctrl Pts',(-11.99999999989,36.03698770308,-3.246220814887));
#9872=CARTESIAN_POINT('Ctrl Pts',(-12.00000000042,36.01653250216,-3.92832252103));
#9873=CARTESIAN_POINT('Ctrl Pts',(-11.99999999844,36.003251535809,-4.54965314868712));
#9874=CARTESIAN_POINT('Ctrl Pts',(-12.00000000337,35.9999999663184,-4.94198226040701));
#9875=CARTESIAN_POINT('Ctrl Pts',(-12.0000000000001,36.0000000049386,-5.1311190912794));
#9876=CARTESIAN_POINT('Origin',(-11.,36.,5.131121190326));
#9877=CARTESIAN_POINT('Origin',(-11.,36.,-5.131119091281));
#9878=CARTESIAN_POINT('Origin',(-12.,37.,-8.));
#9879=CARTESIAN_POINT('',(-12.,36.,8.));
#9880=CARTESIAN_POINT('',(-12.,36.,8.));
#9881=CARTESIAN_POINT('',(-12.,36.,-7.));
#9882=CARTESIAN_POINT('',(-12.,36.00000000494,-5.131124034723));
#9883=CARTESIAN_POINT('',(-12.,6.,-7.));
#9884=CARTESIAN_POINT('',(-12.,6.,-7.));
#9885=CARTESIAN_POINT('',(-12.,5.999999999898,7.));
#9886=CARTESIAN_POINT('',(-12.,6.,-7.));
#9887=CARTESIAN_POINT('',(-12.,5.732050807569,8.));
#9888=CARTESIAN_POINT('Origin',(-12.,4.,7.));
#9889=CARTESIAN_POINT('',(-12.,20.,8.));
#9890=CARTESIAN_POINT('',(-12.,20.,8.));
#9891=CARTESIAN_POINT('',(-12.,20.,7.));
#9892=CARTESIAN_POINT('',(-12.,20.,8.));
#9893=CARTESIAN_POINT('',(-12.,27.,7.));
#9894=CARTESIAN_POINT('',(-12.,20.,7.));
#9895=CARTESIAN_POINT('',(-12.,27.,8.));
#9896=CARTESIAN_POINT('',(-12.,27.,8.));
#9897=CARTESIAN_POINT('',(-12.,36.,8.));
#9898=CARTESIAN_POINT('',(-12.,16.4,2.625));
#9899=CARTESIAN_POINT('Origin',(-12.,16.4,0.));
#9900=CARTESIAN_POINT('Origin',(-12.,16.4,0.));
#9901=CARTESIAN_POINT('',(-6.66390773956619,16.3999999998592,2.625));
#9902=CARTESIAN_POINT('',(-12.,16.4,2.625));
#9903=CARTESIAN_POINT('',(-6.75,15.85786437627,2.56840689250806));
#9904=CARTESIAN_POINT('Ctrl Pts',(-6.66390773956619,16.3999999997184,2.625));
#9905=CARTESIAN_POINT('Ctrl Pts',(-6.72228020467757,16.2208448358157,2.62499999998078));
#9906=CARTESIAN_POINT('Ctrl Pts',(-6.75,16.0334600508686,2.60547137432769));
#9907=CARTESIAN_POINT('Ctrl Pts',(-6.75,15.85786437627,2.56840689250806));
#9908=CARTESIAN_POINT('',(-3.336092260526,16.4,2.625));
#9909=CARTESIAN_POINT('Ctrl Pts',(-6.75,15.85786437627,2.56840689250806));
#9910=CARTESIAN_POINT('Ctrl Pts',(-6.75,15.6110066826013,2.51630052644901));
#9911=CARTESIAN_POINT('Ctrl Pts',(-6.69544690549609,15.3629337030798,2.42419944853985));
#9912=CARTESIAN_POINT('Ctrl Pts',(-6.50091953601999,14.9268772497432,2.18681464246373));
#9913=CARTESIAN_POINT('Ctrl Pts',(-6.36151207057982,14.7383593594213,2.04204903773034));
#9914=CARTESIAN_POINT('Ctrl Pts',(-6.06085872962622,14.4510762985029,1.76929702284452));
#9915=CARTESIAN_POINT('Ctrl Pts',(-5.87839362558371,14.3282234441449,1.61886205539035));
#9916=CARTESIAN_POINT('Ctrl Pts',(-5.57238612680822,14.2004286716704,1.4346071596535));
#9917=CARTESIAN_POINT('Ctrl Pts',(-5.46497331884357,14.1668647431483,1.38050334687473));
#9918=CARTESIAN_POINT('Ctrl Pts',(-5.24008283204397,14.1206143358393,1.30271393580598));
#9919=CARTESIAN_POINT('Ctrl Pts',(-5.12250669020694,14.10786437627,1.27935111772644));
#9920=CARTESIAN_POINT('Ctrl Pts',(-5.,14.10786437627,1.27935111772644));
#9921=CARTESIAN_POINT('Ctrl Pts',(-4.87749330979306,14.10786437627,1.27935111772644));
#9922=CARTESIAN_POINT('Ctrl Pts',(-4.75991716795603,14.1206143358393,1.30271393580598));
#9923=CARTESIAN_POINT('Ctrl Pts',(-4.53502668115643,14.1668647431483,1.38050334687473));
#9924=CARTESIAN_POINT('Ctrl Pts',(-4.42761387319178,14.2004286716704,1.43460715965351));
#9925=CARTESIAN_POINT('Ctrl Pts',(-4.1216063744163,14.3282234441449,1.61886205539036));
#9926=CARTESIAN_POINT('Ctrl Pts',(-3.93914127037378,14.4510762985029,1.76929702284452));
#9927=CARTESIAN_POINT('Ctrl Pts',(-3.63848792942018,14.7383593594213,2.04204903773034));
#9928=CARTESIAN_POINT('Ctrl Pts',(-3.49908046398001,14.9268772497432,2.18681464246373));
#9929=CARTESIAN_POINT('Ctrl Pts',(-3.30455309450391,15.3629337030798,2.42419944853985));
#9930=CARTESIAN_POINT('Ctrl Pts',(-3.25,15.6110066826013,2.51630052644901));
#9931=CARTESIAN_POINT('Ctrl Pts',(-3.25,16.0334600509606,2.60547137434711));
#9932=CARTESIAN_POINT('Ctrl Pts',(-3.2777197953528,16.2208448360119,2.625));
#9933=CARTESIAN_POINT('Ctrl Pts',(-3.33609226052561,16.4000000000001,2.625));
#9934=CARTESIAN_POINT('',(-3.,16.4,2.625));
#9935=CARTESIAN_POINT('',(-12.,16.4,2.625));
#9936=CARTESIAN_POINT('Origin',(-3.,16.4,0.));
#9937=CARTESIAN_POINT('Ctrl Pts',(-3.33609226052562,16.4000000000001,2.625));
#9938=CARTESIAN_POINT('Ctrl Pts',(-3.3492132620138,16.4402706167429,2.625));
#9939=CARTESIAN_POINT('Ctrl Pts',(-3.36382529489561,16.4801444941516,2.62407088270354));
#9940=CARTESIAN_POINT('Ctrl Pts',(-3.46726090935699,16.733454192834,2.61253457823639));
#9941=CARTESIAN_POINT('Ctrl Pts',(-3.59948380965172,16.9291453900179,2.57606325080576));
#9942=CARTESIAN_POINT('Ctrl Pts',(-3.90599376649975,17.2416586072539,2.49181760818345));
#9943=CARTESIAN_POINT('Ctrl Pts',(-4.10241398861631,17.3784789139656,2.43788036890531));
#9944=CARTESIAN_POINT('Ctrl Pts',(-4.53619933463474,17.5616298280266,2.35611948220898));
#9945=CARTESIAN_POINT('Ctrl Pts',(-4.77403581009751,17.60786437627,2.33059834560524));
#9946=CARTESIAN_POINT('Ctrl Pts',(-5.22596418990249,17.60786437627,2.33059834560524));
#9947=CARTESIAN_POINT('Ctrl Pts',(-5.46380066536526,17.5616298280266,2.35611948220898));
#9948=CARTESIAN_POINT('Ctrl Pts',(-5.89758601138369,17.3784789139656,2.43788036890531));
#9949=CARTESIAN_POINT('Ctrl Pts',(-6.09400623350025,17.2416586072539,2.49181760818345));
#9950=CARTESIAN_POINT('Ctrl Pts',(-6.40051619034828,16.9291453900179,2.57606325080576));
#9951=CARTESIAN_POINT('Ctrl Pts',(-6.53273909064301,16.733454192834,2.61253457823639));
#9952=CARTESIAN_POINT('Ctrl Pts',(-6.63617470514179,16.48014449406,2.62407088270771));
#9953=CARTESIAN_POINT('Ctrl Pts',(-6.65078673805434,16.4402706165569,2.62500000000432));
#9954=CARTESIAN_POINT('Ctrl Pts',(-6.66390773956619,16.3999999997184,2.625));
#9955=CARTESIAN_POINT('Origin',(-3.,0.,-8.));
#9956=CARTESIAN_POINT('Origin',(-5.,15.85786437627,8.));
#9957=CARTESIAN_POINT('',(-6.75,15.85786437627,8.));
#9958=CARTESIAN_POINT('',(-6.75,15.85786437627,8.));
#9959=CARTESIAN_POINT('Origin',(-5.,15.85786437627,8.));
#9960=CARTESIAN_POINT('Origin',(0.,0.,8.));
#9961=CARTESIAN_POINT('',(-11.,37.,8.));
#9962=CARTESIAN_POINT('Origin',(-11.,36.,8.));
#9963=CARTESIAN_POINT('',(12.,27.,8.));
#9964=CARTESIAN_POINT('',(-12.,27.,8.));
#9965=CARTESIAN_POINT('',(12.,36.,8.));
#9966=CARTESIAN_POINT('',(12.,27.,8.));
#9967=CARTESIAN_POINT('',(11.,37.,8.));
#9968=CARTESIAN_POINT('Origin',(11.,36.,8.));
#9969=CARTESIAN_POINT('',(6.,37.,8.));
#9970=CARTESIAN_POINT('',(6.,37.,8.));
#9971=CARTESIAN_POINT('',(-2.,30.,8.));
#9972=CARTESIAN_POINT('Origin',(0.,30.,8.));
#9973=CARTESIAN_POINT('Origin',(0.,0.,8.));
#9974=CARTESIAN_POINT('',(12.,5.732050807569,8.));
#9975=CARTESIAN_POINT('',(12.,20.,8.));
#9976=CARTESIAN_POINT('',(12.,5.732050807569,8.));
#9977=CARTESIAN_POINT('',(-12.,20.,8.));
#9978=CARTESIAN_POINT('',(-13.,4.,8.));
#9979=CARTESIAN_POINT('Ctrl Pts',(-13.,4.,8.));
#9980=CARTESIAN_POINT('Ctrl Pts',(-12.722901777919,4.27709822208096,8.));
#9981=CARTESIAN_POINT('Ctrl Pts',(-12.3960872838113,4.61522327220401,8.));
#9982=CARTESIAN_POINT('Ctrl Pts',(-12.0895719998978,5.18473047315088,8.));
#9983=CARTESIAN_POINT('Ctrl Pts',(-12.,5.47717338569331,8.));
#9984=CARTESIAN_POINT('Ctrl Pts',(-12.,5.73205080756888,8.));
#9985=CARTESIAN_POINT('',(-20.,4.,8.));
#9986=CARTESIAN_POINT('',(-13.,4.,8.));
#9987=CARTESIAN_POINT('',(-20.,0.,8.));
#9988=CARTESIAN_POINT('',(-20.,4.,8.));
#9989=CARTESIAN_POINT('',(20.,0.,8.));
#9990=CARTESIAN_POINT('',(-20.,0.,8.));
#9991=CARTESIAN_POINT('',(20.,4.,8.));
#9992=CARTESIAN_POINT('',(20.,0.,8.));
#9993=CARTESIAN_POINT('',(13.,4.,8.));
#9994=CARTESIAN_POINT('',(20.,4.,8.));
#9995=CARTESIAN_POINT('Ctrl Pts',(12.,5.73205080756888,8.));
#9996=CARTESIAN_POINT('Ctrl Pts',(12.,5.47717338569331,8.));
#9997=CARTESIAN_POINT('Ctrl Pts',(12.0895719998978,5.18473047315088,8.));
#9998=CARTESIAN_POINT('Ctrl Pts',(12.3960872838113,4.61522327220401,8.));
#9999=CARTESIAN_POINT('Ctrl Pts',(12.722901777919,4.27709822208096,8.));
#10000=CARTESIAN_POINT('Ctrl Pts',(13.,4.,8.));
#10001=CARTESIAN_POINT('',(3.25,15.85786437627,8.));
#10002=CARTESIAN_POINT('Origin',(5.,15.85786437627,8.));
#10003=CARTESIAN_POINT('Origin',(5.,15.85786437627,8.));
#10004=CARTESIAN_POINT('',(6.75,15.85786437627,2.568406892508));
#10005=CARTESIAN_POINT('',(3.25,15.85786437627,2.56840689250806));
#10006=CARTESIAN_POINT('Ctrl Pts',(6.75,15.85786437627,2.56840689250806));
#10007=CARTESIAN_POINT('Ctrl Pts',(6.75,15.6110066826013,2.51630052644901));
#10008=CARTESIAN_POINT('Ctrl Pts',(6.69544690549608,15.3629337030798,2.42419944853985));
#10009=CARTESIAN_POINT('Ctrl Pts',(6.50091953601999,14.9268772497432,2.18681464246373));
#10010=CARTESIAN_POINT('Ctrl Pts',(6.36151207057982,14.7383593594213,2.04204903773034));
#10011=CARTESIAN_POINT('Ctrl Pts',(6.06085872962622,14.4510762985029,1.76929702284452));
#10012=CARTESIAN_POINT('Ctrl Pts',(5.8783936255837,14.3282234441449,1.61886205539036));
#10013=CARTESIAN_POINT('Ctrl Pts',(5.57238612680822,14.2004286716704,1.43460715965351));
#10014=CARTESIAN_POINT('Ctrl Pts',(5.46497331884357,14.1668647431483,1.38050334687473));
#10015=CARTESIAN_POINT('Ctrl Pts',(5.24008283204397,14.1206143358393,1.30271393580598));
#10016=CARTESIAN_POINT('Ctrl Pts',(5.12250669020694,14.10786437627,1.27935111772644));
#10017=CARTESIAN_POINT('Ctrl Pts',(5.,14.10786437627,1.27935111772644));
#10018=CARTESIAN_POINT('Ctrl Pts',(4.87749330979306,14.10786437627,1.27935111772644));
#10019=CARTESIAN_POINT('Ctrl Pts',(4.75991716795603,14.1206143358393,1.30271393580598));
#10020=CARTESIAN_POINT('Ctrl Pts',(4.53502668115643,14.1668647431483,1.38050334687473));
#10021=CARTESIAN_POINT('Ctrl Pts',(4.42761387319178,14.2004286716704,1.43460715965351));
#10022=CARTESIAN_POINT('Ctrl Pts',(4.1216063744163,14.3282234441449,1.61886205539036));
#10023=CARTESIAN_POINT('Ctrl Pts',(3.93914127037378,14.4510762985029,1.76929702284452));
#10024=CARTESIAN_POINT('Ctrl Pts',(3.63848792942018,14.7383593594213,2.04204903773034));
#10025=CARTESIAN_POINT('Ctrl Pts',(3.49908046398001,14.9268772497432,2.18681464246373));
#10026=CARTESIAN_POINT('Ctrl Pts',(3.30455309450391,15.3629337030798,2.42419944853985));
#10027=CARTESIAN_POINT('Ctrl Pts',(3.25,15.6110066826013,2.51630052644901));
#10028=CARTESIAN_POINT('Ctrl Pts',(3.25,15.85786437627,2.56840689250806));
#10029=CARTESIAN_POINT('',(3.25,15.85786437627,8.));
#10030=CARTESIAN_POINT('',(3.33609226043381,16.3999999998592,2.625));
#10031=CARTESIAN_POINT('Ctrl Pts',(3.25,15.85786437627,2.56840689250806));
#10032=CARTESIAN_POINT('Ctrl Pts',(3.25,16.0334600508686,2.60547137432769));
#10033=CARTESIAN_POINT('Ctrl Pts',(3.27771979532244,16.2208448358157,2.62499999998078));
#10034=CARTESIAN_POINT('Ctrl Pts',(3.33609226043381,16.3999999997184,2.625));
#10035=CARTESIAN_POINT('',(6.66390773956619,16.3999999998592,2.625));
#10036=CARTESIAN_POINT('Ctrl Pts',(3.33609226043381,16.3999999997184,2.625));
#10037=CARTESIAN_POINT('Ctrl Pts',(3.34921326194566,16.4402706165569,2.62500000000432));
#10038=CARTESIAN_POINT('Ctrl Pts',(3.36382529485821,16.48014449406,2.62407088270771));
#10039=CARTESIAN_POINT('Ctrl Pts',(3.46726090935699,16.733454192834,2.61253457823639));
#10040=CARTESIAN_POINT('Ctrl Pts',(3.59948380965172,16.9291453900179,2.57606325080576));
#10041=CARTESIAN_POINT('Ctrl Pts',(3.90599376649975,17.2416586072539,2.49181760818345));
#10042=CARTESIAN_POINT('Ctrl Pts',(4.10241398861631,17.3784789139656,2.43788036890531));
#10043=CARTESIAN_POINT('Ctrl Pts',(4.53619933463474,17.5616298280266,2.35611948220898));
#10044=CARTESIAN_POINT('Ctrl Pts',(4.77403581009751,17.60786437627,2.33059834560524));
#10045=CARTESIAN_POINT('Ctrl Pts',(5.22596418990249,17.60786437627,2.33059834560524));
#10046=CARTESIAN_POINT('Ctrl Pts',(5.46380066536526,17.5616298280266,2.35611948220898));
#10047=CARTESIAN_POINT('Ctrl Pts',(5.89758601138369,17.3784789139656,2.43788036890531));
#10048=CARTESIAN_POINT('Ctrl Pts',(6.09400623350025,17.2416586072539,2.49181760818345));
#10049=CARTESIAN_POINT('Ctrl Pts',(6.40051619034828,16.9291453900179,2.57606325080576));
#10050=CARTESIAN_POINT('Ctrl Pts',(6.53273909064301,16.733454192834,2.61253457823639));
#10051=CARTESIAN_POINT('Ctrl Pts',(6.63617470514179,16.48014449406,2.62407088270771));
#10052=CARTESIAN_POINT('Ctrl Pts',(6.65078673805434,16.4402706165569,2.62500000000432));
#10053=CARTESIAN_POINT('Ctrl Pts',(6.66390773956619,16.3999999997184,2.625));
#10054=CARTESIAN_POINT('Ctrl Pts',(6.66390773956619,16.3999999997184,2.625));
#10055=CARTESIAN_POINT('Ctrl Pts',(6.72228020467757,16.2208448358157,2.62499999998078));
#10056=CARTESIAN_POINT('Ctrl Pts',(6.75,16.0334600508686,2.60547137432769));
#10057=CARTESIAN_POINT('Ctrl Pts',(6.75,15.85786437627,2.56840689250806));
#10058=CARTESIAN_POINT('Origin',(12.,16.4,0.));
#10059=CARTESIAN_POINT('',(3.,16.4,2.625));
#10060=CARTESIAN_POINT('Origin',(3.,16.4,0.));
#10061=CARTESIAN_POINT('',(12.,16.4,2.625));
#10062=CARTESIAN_POINT('',(12.,16.4,2.625));
#10063=CARTESIAN_POINT('',(12.,16.4,2.625));
#10064=CARTESIAN_POINT('Origin',(12.,16.4,0.));
#10065=CARTESIAN_POINT('Origin',(12.,5.,-8.));
#10066=CARTESIAN_POINT('',(12.,6.,-7.));
#10067=CARTESIAN_POINT('',(12.,5.999999999485,7.));
#10068=CARTESIAN_POINT('',(12.,6.,-7.));
#10069=CARTESIAN_POINT('',(12.,36.,-7.));
#10070=CARTESIAN_POINT('',(12.,36.,-7.));
#10071=CARTESIAN_POINT('',(12.,36.,-5.13112138723605));
#10072=CARTESIAN_POINT('',(12.,36.,-5.131121557209));
#10073=CARTESIAN_POINT('',(11.9999999999999,36.10888778104,-0.00016660306200075));
#10074=CARTESIAN_POINT('Ctrl Pts',(12.,36.10888778104,-0.0001666008893355));
#10075=CARTESIAN_POINT('Ctrl Pts',(12.,36.10888720385,-0.2115948044887));
#10076=CARTESIAN_POINT('Ctrl Pts',(12.,36.10647748554,-0.632542946972));
#10077=CARTESIAN_POINT('Ctrl Pts',(12.,36.09662552275,-1.246846637783));
#10078=CARTESIAN_POINT('Ctrl Pts',(12.,36.08098057782,-1.878213676881));
#10079=CARTESIAN_POINT('Ctrl Pts',(12.,36.06231044761,-2.484098080739));
#10080=CARTESIAN_POINT('Ctrl Pts',(12.,36.04274891785,-3.075021505576));
#10081=CARTESIAN_POINT('Ctrl Pts',(12.,36.02306872989,-3.696652254043));
#10082=CARTESIAN_POINT('Ctrl Pts',(12.,36.0059704833598,-4.37191141631148));
#10083=CARTESIAN_POINT('Ctrl Pts',(12.,35.9999999979788,-4.87066496985907));
#10084=CARTESIAN_POINT('Ctrl Pts',(12.,36.,-5.13112138723605));
#10085=CARTESIAN_POINT('',(12.,36.0000000210414,5.1311211680071));
#10086=CARTESIAN_POINT('Ctrl Pts',(11.9999999999999,36.00000002104,5.13112116800713));
#10087=CARTESIAN_POINT('Ctrl Pts',(11.99999997181,36.0000000085565,4.8397925008905));
#10088=CARTESIAN_POINT('Ctrl Pts',(12.00000001305,36.0075844610583,4.27293018632732));
#10089=CARTESIAN_POINT('Ctrl Pts',(11.99999999661,36.0287089676,3.502562898396));
#10090=CARTESIAN_POINT('Ctrl Pts',(12.00000000053,36.05480007394,2.714420520144));
#10091=CARTESIAN_POINT('Ctrl Pts',(12.00000000128,36.08110280775,1.891087904674));
#10092=CARTESIAN_POINT('Ctrl Pts',(11.99999999435,36.1023071011,1.013181682868));
#10093=CARTESIAN_POINT('Ctrl Pts',(12.00000001234,36.10888952645,0.3484660678232));
#10094=CARTESIAN_POINT('Ctrl Pts',(12.,36.10888778104,-0.0001666008893355));
#10095=CARTESIAN_POINT('',(12.,36.,8.));
#10096=CARTESIAN_POINT('',(12.,27.,7.));
#10097=CARTESIAN_POINT('',(12.,27.,8.));
#10098=CARTESIAN_POINT('',(12.,20.,7.));
#10099=CARTESIAN_POINT('',(12.,20.,7.));
#10100=CARTESIAN_POINT('',(12.,20.,8.));
#10101=CARTESIAN_POINT('Origin',(12.,4.,7.));
#10102=CARTESIAN_POINT('Origin',(3.,0.,-8.));
#10103=CARTESIAN_POINT('Origin',(13.,6.,-43.78380184031));
#10104=CARTESIAN_POINT('',(13.,5.,7.));
#10105=CARTESIAN_POINT('Origin',(13.,6.,7.));
#10106=CARTESIAN_POINT('',(13.,5.,0.));
#10107=CARTESIAN_POINT('',(13.,5.,0.));
#10108=CARTESIAN_POINT('',(13.,5.,-7.));
#10109=CARTESIAN_POINT('',(13.,5.,-7.));
#10110=CARTESIAN_POINT('Origin',(13.,6.,-7.));
#10111=CARTESIAN_POINT('Origin',(13.,6.,-7.));
#10112=CARTESIAN_POINT('',(11.,6.,-8.));
#10113=CARTESIAN_POINT('',(13.,4.,-8.));
#10114=CARTESIAN_POINT('Origin',(13.,6.,-8.));
#10115=CARTESIAN_POINT('Origin',(11.,6.,-7.));
#10116=CARTESIAN_POINT('Origin',(13.,4.,-7.));
#10117=CARTESIAN_POINT('Origin',(0.,0.,-8.));
#10118=CARTESIAN_POINT('',(-11.,6.,-8.));
#10119=CARTESIAN_POINT('',(-11.,37.,-8.));
#10120=CARTESIAN_POINT('',(-11.,6.,-8.));
#10121=CARTESIAN_POINT('',(6.,37.,-8.));
#10122=CARTESIAN_POINT('',(11.,37.,-8.));
#10123=CARTESIAN_POINT('',(6.,37.,-8.));
#10124=CARTESIAN_POINT('',(11.,37.,-8.));
#10125=CARTESIAN_POINT('',(20.,4.,-8.));
#10126=CARTESIAN_POINT('',(13.,4.,-8.));
#10127=CARTESIAN_POINT('',(20.,0.,-8.));
#10128=CARTESIAN_POINT('',(20.,4.,-8.));
#10129=CARTESIAN_POINT('',(-20.,0.,-8.));
#10130=CARTESIAN_POINT('',(-20.,0.,-8.));
#10131=CARTESIAN_POINT('',(-20.,4.,-8.));
#10132=CARTESIAN_POINT('',(-20.,0.,-8.));
#10133=CARTESIAN_POINT('',(-13.,4.,-8.));
#10134=CARTESIAN_POINT('',(-20.,4.,-8.));
#10135=CARTESIAN_POINT('Origin',(-13.,6.,-8.));
#10136=CARTESIAN_POINT('',(-2.,30.,-8.));
#10137=CARTESIAN_POINT('Origin',(0.,30.,-8.));
#10138=CARTESIAN_POINT('Origin',(0.,30.,-8.));
#10139=CARTESIAN_POINT('',(-2.,30.,-8.));
#10140=CARTESIAN_POINT('Origin',(-11.,-152.5212,-7.));
#10141=CARTESIAN_POINT('Origin',(-11.,6.,-7.));
#10142=CARTESIAN_POINT('Origin',(-11.,36.,-7.));
#10143=CARTESIAN_POINT('Origin',(-11.,36.,8.15648));
#10144=CARTESIAN_POINT('',(-11.00000012291,37.,-5.131119600082));
#10145=CARTESIAN_POINT('Origin',(12.,37.,-8.));
#10146=CARTESIAN_POINT('',(-11.,37.,8.));
#10147=CARTESIAN_POINT('Origin',(12.,37.,-8.));
#10148=CARTESIAN_POINT('Origin',(12.,37.,-8.));
#10149=CARTESIAN_POINT('',(11.,37.,8.));
#10150=CARTESIAN_POINT('Origin',(12.,37.,-8.));
#10151=CARTESIAN_POINT('',(11.00000000411,37.,-5.131121402775));
#10152=CARTESIAN_POINT('Origin',(-11.,36.,43.78380184031));
#10153=CARTESIAN_POINT('Origin',(11.,36.,43.78380184031));
#10154=CARTESIAN_POINT('Origin',(11.,36.,5.131121166588));
#10155=CARTESIAN_POINT('Ctrl Pts',(10.87639820398,36.99238627919,5.190418362005));
#10156=CARTESIAN_POINT('Ctrl Pts',(10.87769651652,36.99251157435,5.170658557952));
#10157=CARTESIAN_POINT('Ctrl Pts',(10.89692694025,36.99460171349,4.877137850237));
#10158=CARTESIAN_POINT('Ctrl Pts',(10.9315020989,37.0047000695,4.325352885477));
#10159=CARTESIAN_POINT('Ctrl Pts',(10.97577779548,37.02831631823,3.528331623006));
#10160=CARTESIAN_POINT('Ctrl Pts',(11.01326259241,37.05497526794,2.729327118972));
#10161=CARTESIAN_POINT('Ctrl Pts',(11.04382137072,37.08079008034,1.88909513595));
#10162=CARTESIAN_POINT('Ctrl Pts',(11.06541962492,37.10108731992,0.9746583446556));
#10163=CARTESIAN_POINT('Ctrl Pts',(11.07091432789,37.10655625449,0.3159910511012));
#10164=CARTESIAN_POINT('Ctrl Pts',(11.07072948767,37.10637175836,-0.04163617506052));
#10165=CARTESIAN_POINT('Ctrl Pts',(11.07070810544,37.10635038289,-0.06236933689121));
#10166=CARTESIAN_POINT('Ctrl Pts',(11.57504126409,37.07940693165,5.190257582826));
#10167=CARTESIAN_POINT('Ctrl Pts',(11.57645336605,37.07861826856,5.170553848682));
#10168=CARTESIAN_POINT('Ctrl Pts',(11.59734297401,37.06717003218,4.87782845147));
#10169=CARTESIAN_POINT('Ctrl Pts',(11.63415546378,37.0529119173,4.326540263707));
#10170=CARTESIAN_POINT('Ctrl Pts',(11.67980309249,37.04535955746,3.528923029992));
#10171=CARTESIAN_POINT('Ctrl Pts',(11.71737756968,37.04564363316,2.72899893329));
#10172=CARTESIAN_POINT('Ctrl Pts',(11.74726727952,37.04995202718,1.888155892492));
#10173=CARTESIAN_POINT('Ctrl Pts',(11.76797944015,37.05503499255,0.9738259564121));
#10174=CARTESIAN_POINT('Ctrl Pts',(11.77318315821,37.05662938656,0.3157193840525));
#10175=CARTESIAN_POINT('Ctrl Pts',(11.77300787451,37.05657527129,-0.04160039065528));
#10176=CARTESIAN_POINT('Ctrl Pts',(11.77298757863,37.0565689799,-0.06231576499393));
#10177=CARTESIAN_POINT('Ctrl Pts',(12.0748185662,36.58352740788,5.191173770148));
#10178=CARTESIAN_POINT('Ctrl Pts',(12.07558184615,36.58208430631,5.171161356908));
#10179=CARTESIAN_POINT('Ctrl Pts',(12.08684498807,36.56096809879,4.873900518236));
#10180=CARTESIAN_POINT('Ctrl Pts',(12.10588924084,36.53002481672,4.315495143085));
#10181=CARTESIAN_POINT('Ctrl Pts',(12.12786170733,36.50231553734,3.511843211855));
#10182=CARTESIAN_POINT('Ctrl Pts',(12.14473054851,36.48628864437,2.710134870967));
#10183=CARTESIAN_POINT('Ctrl Pts',(12.15728217879,36.47775237489,1.87171629668));
#10184=CARTESIAN_POINT('Ctrl Pts',(12.16548507289,36.47397603557,0.9640221888825));
#10185=CARTESIAN_POINT('Ctrl Pts',(12.16746589788,36.47334779007,0.3125390240587));
#10186=CARTESIAN_POINT('Ctrl Pts',(12.16739888806,36.47336841638,-0.04118134654457));
#10187=CARTESIAN_POINT('Ctrl Pts',(12.16739110543,36.47337076861,-0.06168816472244));
#10188=CARTESIAN_POINT('Ctrl Pts',(11.9932691391,35.88422585437,5.192465799906));
#10189=CARTESIAN_POINT('Ctrl Pts',(11.99311750496,35.8828886515,5.172016179191));
#10190=CARTESIAN_POINT('Ctrl Pts',(11.99083530679,35.86337341576,4.86835995167));
#10191=CARTESIAN_POINT('Ctrl Pts',(11.98570312504,35.83618480774,4.300669943404));
#10192=CARTESIAN_POINT('Ctrl Pts',(11.97707105556,35.8147556383,3.490162717829));
#10193=CARTESIAN_POINT('Ctrl Pts',(11.96828419718,35.80496385934,2.687170896915));
#10194=CARTESIAN_POINT('Ctrl Pts',(11.9600969239,35.80207422425,1.852356959427));
#10195=CARTESIAN_POINT('Ctrl Pts',(11.95374025469,35.80257324593,0.9527495005316));
#10196=CARTESIAN_POINT('Ctrl Pts',(11.95203263857,35.80307516529,0.3088837822729));
#10197=CARTESIAN_POINT('Ctrl Pts',(11.95208976203,35.80305769695,-0.04069972159253));
#10198=CARTESIAN_POINT('Ctrl Pts',(11.95209634362,35.80305563768,-0.06096681520975));
#10199=CARTESIAN_POINT('Origin',(11.,36.10888778108,-0.0001666050799347));
#10200=CARTESIAN_POINT('Ctrl Pts',(10.88028304336,37.1015617965,0.123806950294));
#10201=CARTESIAN_POINT('Ctrl Pts',(10.88028304336,37.10165143422,0.08248224247726));
#10202=CARTESIAN_POINT('Ctrl Pts',(10.88028304336,37.1019259464,-0.1723252126584));
#10203=CARTESIAN_POINT('Ctrl Pts',(10.88028304336,37.09933054386,-0.6372922628576));
#10204=CARTESIAN_POINT('Ctrl Pts',(10.88028304336,37.08914764459,-1.271464818044));
#10205=CARTESIAN_POINT('Ctrl Pts',(10.88028304336,37.07366901929,-1.89602670484));
#10206=CARTESIAN_POINT('Ctrl Pts',(10.88028304336,37.05480294858,-2.51029661392));
#10207=CARTESIAN_POINT('Ctrl Pts',(10.88028304336,37.03456745556,-3.12121065189));
#10208=CARTESIAN_POINT('Ctrl Pts',(10.88028304336,37.01469479526,-3.751183702533));
#10209=CARTESIAN_POINT('Ctrl Pts',(10.88028304336,36.99796087928,-4.424629516724));
#10210=CARTESIAN_POINT('Ctrl Pts',(10.88028304336,36.99258729792,-4.908935980834));
#10211=CARTESIAN_POINT('Ctrl Pts',(10.88028304336,36.99282614041,-5.170754488191));
#10212=CARTESIAN_POINT('Ctrl Pts',(10.88028304336,36.99286279613,-5.190561784574));
#10213=CARTESIAN_POINT('Ctrl Pts',(11.57926121074,37.18584731036,0.1239869276598));
#10214=CARTESIAN_POINT('Ctrl Pts',(11.57926121074,37.18593708415,0.08260222517352));
#10215=CARTESIAN_POINT('Ctrl Pts',(11.57926121074,37.18621200725,-0.1725758878834));
#10216=CARTESIAN_POINT('Ctrl Pts',(11.57926121074,37.18361272676,-0.638219248976));
#10217=CARTESIAN_POINT('Ctrl Pts',(11.57926121074,37.17341622784,-1.273216845643));
#10218=CARTESIAN_POINT('Ctrl Pts',(11.57926121074,37.15792160269,-1.898406858163));
#10219=CARTESIAN_POINT('Ctrl Pts',(11.57926121074,37.13904415592,-2.513037048283));
#10220=CARTESIAN_POINT('Ctrl Pts',(11.57926121074,37.11880713331,-3.123995722929));
#10221=CARTESIAN_POINT('Ctrl Pts',(11.57926121074,37.0989454502,-3.75363319921));
#10222=CARTESIAN_POINT('Ctrl Pts',(11.57926121074,37.08223377732,-4.426235196415));
#10223=CARTESIAN_POINT('Ctrl Pts',(11.57926121074,37.07687356091,-4.90952025416));
#10224=CARTESIAN_POINT('Ctrl Pts',(11.57926121074,37.0771118124,-5.170651184102));
#10225=CARTESIAN_POINT('Ctrl Pts',(11.57926121074,37.07714837518,-5.190405681367));
#10226=CARTESIAN_POINT('Ctrl Pts',(12.0770937892,36.68801592067,0.1229238934798));
#10227=CARTESIAN_POINT('Ctrl Pts',(12.0770937892,36.68810489079,0.08189354879861));
#10228=CARTESIAN_POINT('Ctrl Pts',(12.0770937892,36.68837738675,-0.1710952776352));
#10229=CARTESIAN_POINT('Ctrl Pts',(12.0770937892,36.68580101136,-0.632744016443));
#10230=CARTESIAN_POINT('Ctrl Pts',(12.0770937892,36.6756848386,-1.262868515376));
#10231=CARTESIAN_POINT('Ctrl Pts',(12.0770937892,36.66028471638,-1.884348510744));
#10232=CARTESIAN_POINT('Ctrl Pts',(12.0770937892,36.64147446212,-2.496850705164));
#10233=CARTESIAN_POINT('Ctrl Pts',(12.0770937892,36.62124647408,-3.107545733809));
#10234=CARTESIAN_POINT('Ctrl Pts',(12.0770937892,36.60131995433,-3.739165276085));
#10235=CARTESIAN_POINT('Ctrl Pts',(12.0770937892,36.58447690284,-4.416751268335));
#10236=CARTESIAN_POINT('Ctrl Pts',(12.0770937892,36.57903774649,-4.906069250679));
#10237=CARTESIAN_POINT('Ctrl Pts',(12.0770937892,36.57927948871,-5.171261348479));
#10238=CARTESIAN_POINT('Ctrl Pts',(12.0770937892,36.57931660044,-5.19132770311));
#10239=CARTESIAN_POINT('Ctrl Pts',(11.9928080612,35.98903943522,0.1214313481916));
#10240=CARTESIAN_POINT('Ctrl Pts',(11.9928080612,35.98912727695,0.0808985369691));
#10241=CARTESIAN_POINT('Ctrl Pts',(11.9928080612,35.98939636512,-0.1690164377528));
#10242=CARTESIAN_POINT('Ctrl Pts',(11.9928080612,35.98685214946,-0.6250565566483));
#10243=CARTESIAN_POINT('Ctrl Pts',(11.9928080612,35.97684875804,-1.248339018703));
#10244=CARTESIAN_POINT('Ctrl Pts',(11.9928080612,35.96158132197,-1.864609991895));
#10245=CARTESIAN_POINT('Ctrl Pts',(11.9928080612,35.94286540886,-2.474124389668));
#10246=CARTESIAN_POINT('Ctrl Pts',(11.9928080612,35.92265010573,-3.084449248094));
#10247=CARTESIAN_POINT('Ctrl Pts',(11.9928080612,35.90263255259,-3.718851695488));
#10248=CARTESIAN_POINT('Ctrl Pts',(11.9928080612,35.88560503994,-4.403435429169));
#10249=CARTESIAN_POINT('Ctrl Pts',(11.9928080612,35.88005504854,-4.901223894733));
#10250=CARTESIAN_POINT('Ctrl Pts',(11.9928080612,35.8803016919,-5.172118045266));
#10251=CARTESIAN_POINT('Ctrl Pts',(11.9928080612,35.88033957438,-5.192622260927));
#10252=CARTESIAN_POINT('Origin',(11.,36.,-5.131121385248));
#10253=CARTESIAN_POINT('Origin',(11.,36.,8.15648));
#10254=CARTESIAN_POINT('Origin',(11.,36.,-7.));
#10255=CARTESIAN_POINT('Origin',(11.,266.1186496051,-7.));
#10256=CARTESIAN_POINT('Origin',(-13.,6.,-7.));
#10257=CARTESIAN_POINT('',(-13.,5.,-7.));
#10258=CARTESIAN_POINT('Origin',(-13.,4.,-7.));
#10259=CARTESIAN_POINT('Origin',(-13.,6.,-7.));
#10260=CARTESIAN_POINT('Origin',(-13.,6.,-43.78380184031));
#10261=CARTESIAN_POINT('',(-13.,5.,0.));
#10262=CARTESIAN_POINT('',(-13.,5.,-7.));
#10263=CARTESIAN_POINT('',(-13.,5.,7.));
#10264=CARTESIAN_POINT('',(-13.,5.,-1.571160412673E-14));
#10265=CARTESIAN_POINT('Origin',(-13.,6.,7.));
#10266=CARTESIAN_POINT('Origin',(-12.,5.,-8.));
#10267=CARTESIAN_POINT('',(-17.,5.,2.44929359829471E-16));
#10268=CARTESIAN_POINT('Origin',(-15.,5.,0.));
#10269=CARTESIAN_POINT('',(-20.,5.,-7.));
#10270=CARTESIAN_POINT('',(-20.,5.,-7.));
#10271=CARTESIAN_POINT('',(-20.,5.,7.));
#10272=CARTESIAN_POINT('',(-20.,5.,7.));
#10273=CARTESIAN_POINT('',(-13.,5.,7.));
#10274=CARTESIAN_POINT('Origin',(-15.,5.,0.));
#10275=CARTESIAN_POINT('Origin',(-15.,5.,0.));
#10276=CARTESIAN_POINT('',(-17.,0.,0.));
#10277=CARTESIAN_POINT('Origin',(-15.,0.,0.));
#10278=CARTESIAN_POINT('',(-17.,5.,2.44929359829471E-16));
#10279=CARTESIAN_POINT('Origin',(-21.,0.,-8.));
#10280=CARTESIAN_POINT('',(-21.,0.,7.));
#10281=CARTESIAN_POINT('Origin',(-20.,0.,7.));
#10282=CARTESIAN_POINT('',(-21.,0.,-7.));
#10283=CARTESIAN_POINT('',(-21.,0.,-7.));
#10284=CARTESIAN_POINT('Origin',(-20.,0.,-7.));
#10285=CARTESIAN_POINT('',(21.,0.,-7.));
#10286=CARTESIAN_POINT('Origin',(20.,0.,-7.));
#10287=CARTESIAN_POINT('',(21.,0.,7.));
#10288=CARTESIAN_POINT('',(21.,0.,-7.));
#10289=CARTESIAN_POINT('Origin',(20.,0.,7.));
#10290=CARTESIAN_POINT('',(13.,0.,0.));
#10291=CARTESIAN_POINT('Origin',(15.,0.,0.));
#10292=CARTESIAN_POINT('Origin',(15.,5.,0.));
#10293=CARTESIAN_POINT('',(13.,5.,2.44929359829471E-16));
#10294=CARTESIAN_POINT('Origin',(15.,5.,0.));
#10295=CARTESIAN_POINT('Origin',(21.,5.,-8.));
#10296=CARTESIAN_POINT('',(20.,5.,7.));
#10297=CARTESIAN_POINT('',(20.,5.,7.));
#10298=CARTESIAN_POINT('',(20.,5.,-7.));
#10299=CARTESIAN_POINT('',(20.,5.,7.));
#10300=CARTESIAN_POINT('',(13.,5.,-7.));
#10301=CARTESIAN_POINT('Origin',(-75.7512,4.,-7.));
#10302=CARTESIAN_POINT('Origin',(20.,4.,-7.));
#10303=CARTESIAN_POINT('Origin',(20.,4.,-7.));
#10304=CARTESIAN_POINT('',(21.,4.,-7.));
#10305=CARTESIAN_POINT('Origin',(20.,4.,-7.));
#10306=CARTESIAN_POINT('Origin',(20.,4.,-7.));
#10307=CARTESIAN_POINT('Origin',(20.,243.2441960567,-7.));
#10308=CARTESIAN_POINT('',(21.,4.,-7.));
#10309=CARTESIAN_POINT('Origin',(21.,0.,-8.));
#10310=CARTESIAN_POINT('',(21.,4.,7.));
#10311=CARTESIAN_POINT('',(21.,0.,7.));
#10312=CARTESIAN_POINT('',(21.,4.,7.));
#10313=CARTESIAN_POINT('Origin',(20.,-152.5212,7.));
#10314=CARTESIAN_POINT('Origin',(20.,4.,7.));
#10315=CARTESIAN_POINT('Origin',(20.,4.,7.));
#10316=CARTESIAN_POINT('Origin',(20.,4.,7.));
#10317=CARTESIAN_POINT('Origin',(20.,4.,7.));
#10318=CARTESIAN_POINT('Origin',(75.7512,4.,7.));
#10319=CARTESIAN_POINT('Origin',(13.,4.,7.));
#10320=CARTESIAN_POINT('Origin',(13.,4.,7.));
#10321=CARTESIAN_POINT('Origin',(20.,4.,43.78380184031));
#10322=CARTESIAN_POINT('Origin',(-20.,257.4707560608,7.));
#10323=CARTESIAN_POINT('',(-21.,4.,7.));
#10324=CARTESIAN_POINT('Origin',(-20.,4.,7.));
#10325=CARTESIAN_POINT('',(-21.,4.,7.));
#10326=CARTESIAN_POINT('Origin',(-21.,5.,-8.));
#10327=CARTESIAN_POINT('',(-21.,4.,-7.));
#10328=CARTESIAN_POINT('',(-21.,4.,7.));
#10329=CARTESIAN_POINT('',(-21.,0.,-7.));
#10330=CARTESIAN_POINT('Origin',(-20.,-152.5212,-7.));
#10331=CARTESIAN_POINT('Origin',(-20.,4.,-7.));
#10332=CARTESIAN_POINT('Origin',(-20.,4.,-7.));
#10333=CARTESIAN_POINT('Origin',(-20.,4.,-7.));
#10334=CARTESIAN_POINT('Origin',(-20.,4.,-7.));
#10335=CARTESIAN_POINT('Origin',(-75.7512,4.,-7.));
#10336=CARTESIAN_POINT('Origin',(-20.,4.,43.78380184031));
#10337=CARTESIAN_POINT('Origin',(-20.,4.,7.));
#10338=CARTESIAN_POINT('Origin',(-20.,4.,7.));
#10339=CARTESIAN_POINT('Origin',(-20.,4.,7.));
#10340=CARTESIAN_POINT('Origin',(75.7512,4.,7.));
#10341=CARTESIAN_POINT('Origin',(-13.,4.,7.));
#10342=CARTESIAN_POINT('Origin',(-13.,4.,7.));
#10343=CARTESIAN_POINT('Origin',(-21.1,20.,8.));
#10344=CARTESIAN_POINT('',(-12.,20.,7.));
#10345=CARTESIAN_POINT('Origin',(-21.1,20.,7.));
#10346=CARTESIAN_POINT('',(-12.,27.,7.));
#10347=CARTESIAN_POINT('Origin',(-21.1,27.,7.));
#10348=CARTESIAN_POINT('Origin',(-12.,16.4,0.));
#10349=CARTESIAN_POINT('',(-12.,19.4,-3.67394039744206E-16));
#10350=CARTESIAN_POINT('Origin',(-12.,16.4,0.));
#10351=CARTESIAN_POINT('',(-8.,19.4,-3.67394039744206E-16));
#10352=CARTESIAN_POINT('',(-12.,19.4,-3.67394039744206E-16));
#10353=CARTESIAN_POINT('Origin',(-8.,16.4,0.));
#10354=CARTESIAN_POINT('Origin',(-8.,16.4,0.));
#10355=CARTESIAN_POINT('',(-8.,13.775,0.));
#10356=CARTESIAN_POINT('Origin',(-8.,16.4,0.));
#10357=CARTESIAN_POINT('Origin',(12.,16.4,0.));
#10358=CARTESIAN_POINT('',(12.,13.4,-3.67394039744206E-16));
#10359=CARTESIAN_POINT('Origin',(12.,16.4,0.));
#10360=CARTESIAN_POINT('',(8.,13.4,-3.67394039744206E-16));
#10361=CARTESIAN_POINT('',(12.,13.4,-3.67394039744206E-16));
#10362=CARTESIAN_POINT('Origin',(8.,16.4,0.));
#10363=CARTESIAN_POINT('Origin',(8.,16.4,0.));
#10364=CARTESIAN_POINT('',(8.,19.025,0.));
#10365=CARTESIAN_POINT('Origin',(8.,16.4,0.));
#17072=UNCERTAINTY_MEASURE_WITH_UNIT(LENGTH_MEASURE(0.01),#17114,
'DISTANCE_ACCURACY_VALUE',
'Maximum model space distance between geometric entities at asserted c
onnectivities');
#17090=UNCERTAINTY_MEASURE_WITH_UNIT(LENGTH_MEASURE(0.01),#17114,
'DISTANCE_ACCURACY_VALUE',
'Maximum model space distance between geometric entities at asserted c
onnectivities');
#17095=(
GEOMETRIC_REPRESENTATION_CONTEXT(3)
GLOBAL_UNCERTAINTY_ASSIGNED_CONTEXT((#17072))
GLOBAL_UNIT_ASSIGNED_CONTEXT((#17114,#17116,#17117))
REPRESENTATION_CONTEXT('','3D')
);
#17113=(
GEOMETRIC_REPRESENTATION_CONTEXT(3)
GLOBAL_UNCERTAINTY_ASSIGNED_CONTEXT((#17090))
GLOBAL_UNIT_ASSIGNED_CONTEXT((#17114,#17116,#17117))
REPRESENTATION_CONTEXT('','3D')
);
#17114=(
LENGTH_UNIT()
NAMED_UNIT(*)
SI_UNIT(.MILLI.,.METRE.)
);
#17116=(
NAMED_UNIT(*)
PLANE_ANGLE_UNIT()
SI_UNIT($,.RADIAN.)
);
#17117=(
NAMED_UNIT(*)
SI_UNIT($,.STERADIAN.)
SOLID_ANGLE_UNIT()
);
#17122=SHAPE_DEFINITION_REPRESENTATION(#17144,#17188);
#17144=PRODUCT_DEFINITION_SHAPE('',$,#17211);
#17188=SHAPE_REPRESENTATION('',(#6301,#241,#242),#17095);
#17206=PRODUCT_DEFINITION_CONTEXT('part definition',#17274,'design');
#17211=PRODUCT_DEFINITION('COLUMN','COLUMN',#17233,#17206);
#17233=PRODUCT_DEFINITION_FORMATION('',$,#17280);
#17274=APPLICATION_CONTEXT(
'Core Data for Automotive Mechanical Design Process');
#17275=PRODUCT_CONTEXT('part definition',#17274,'mechanical');
#17280=PRODUCT('COLUMN','COLUMN','NOT SPECIFIED',(#17275));
#17298=PRESENTATION_STYLE_ASSIGNMENT((#17299));
#17299=SURFACE_STYLE_USAGE(.BOTH.,#17300);
#17300=SURFACE_SIDE_STYLE('',(#17301));
#17301=SURFACE_STYLE_FILL_AREA(#17302);
#17302=FILL_AREA_STYLE('Steel - Satin',(#17303));
#17303=FILL_AREA_STYLE_COLOUR('Steel - Satin',#17304);
#17304=COLOUR_RGB('Steel - Satin', 0.09019608, 0.27058824, 0.51372549);
ENDSEC;
END-ISO-10303-21;
